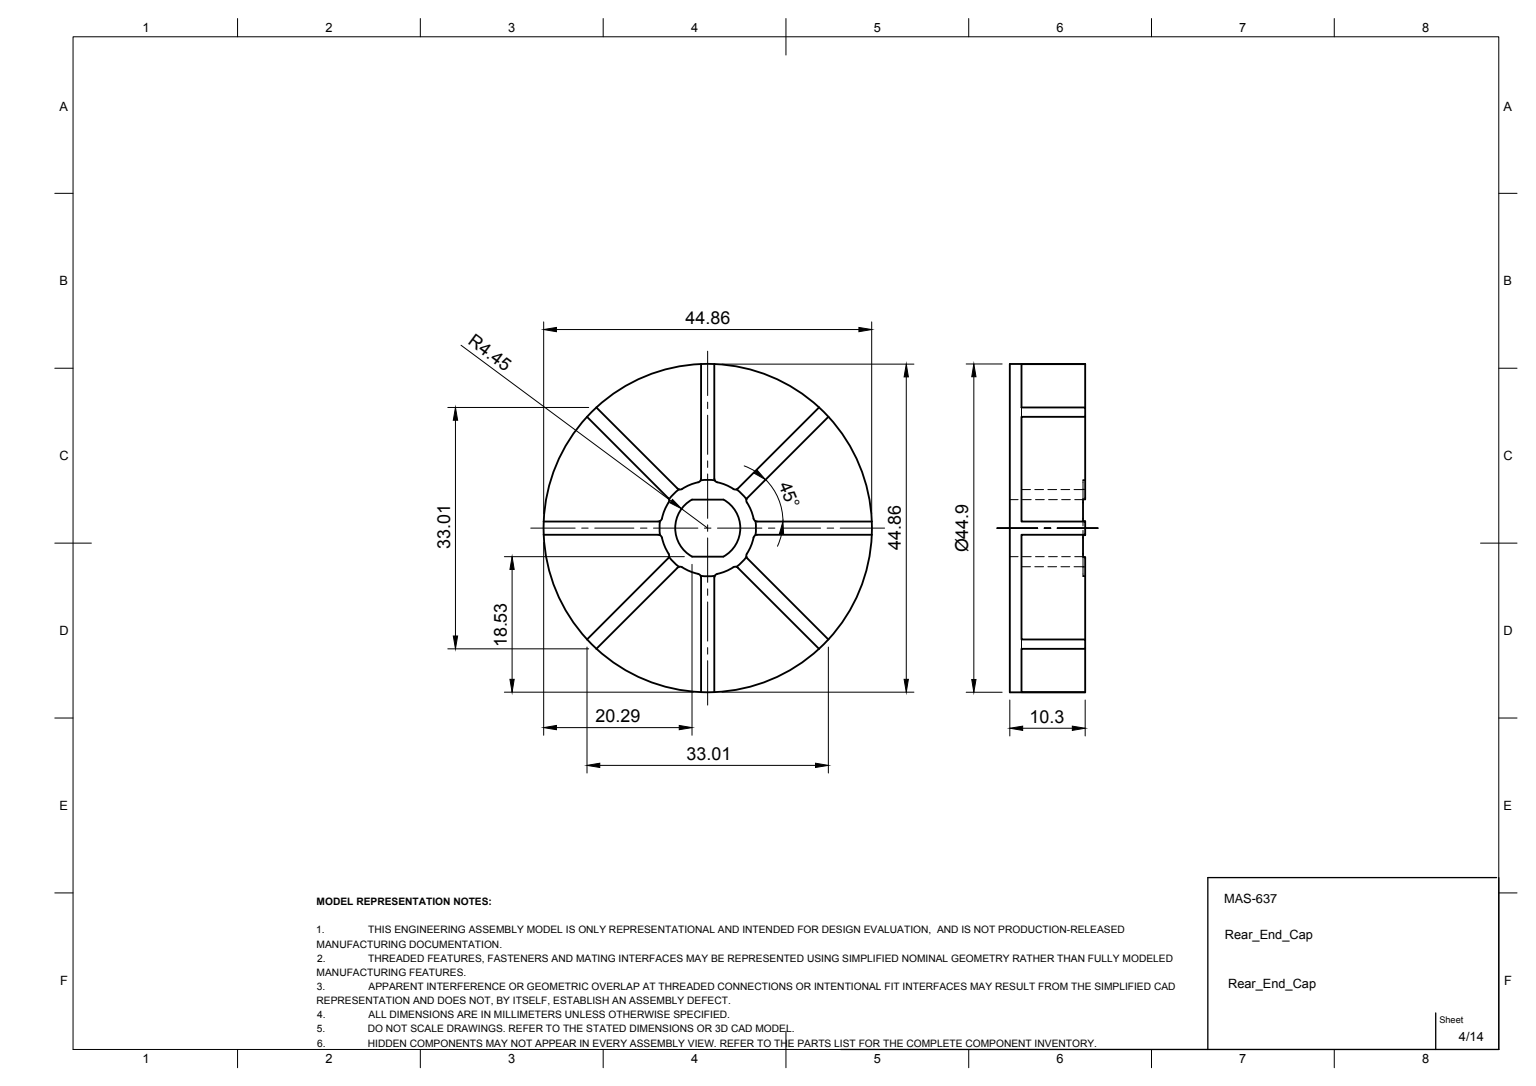
ISO-10303-21;
HEADER;
FILE_DESCRIPTION((''),'2;1');
FILE_NAME('Rear_End_Cap.step','2026-10-09T10:11:57-07:00',(''),(''),'','','');
FILE_SCHEMA (('AUTOMOTIVE_DESIGN { 1 0 10303 214 3 1 1 }'));
ENDSEC;
DATA;
#10=MECHANICAL_DESIGN_GEOMETRIC_PRESENTATION_REPRESENTATION('',(#124),#13510);
#94=SHAPE_REPRESENTATION_RELATIONSHIP('SRR','None',#13564,#109) ;
#109=ADVANCED_BREP_SHAPE_REPRESENTATION('',(#156),#13496) ;
#124=STYLED_ITEM('',(#13648),#156) ;
#156=MANIFOLD_SOLID_BREP('Body1',#7373) ;
#215=FACE_BOUND('',#1218,.T.) ;
#216=FACE_BOUND('',#1281,.T.) ;
#288=PLANE('',#7723) ;
#289=PLANE('',#7727) ;
#290=PLANE('',#7746) ;
#291=PLANE('',#7747) ;
#292=PLANE('',#7751) ;
#293=PLANE('',#7752) ;
#294=PLANE('',#7753) ;
#295=PLANE('',#7756) ;
#296=PLANE('',#7760) ;
#297=PLANE('',#7761) ;
#298=PLANE('',#7762) ;
#299=PLANE('',#7763) ;
#300=PLANE('',#7766) ;
#301=PLANE('',#7769) ;
#302=PLANE('',#7860) ;
#303=PLANE('',#7861) ;
#304=PLANE('',#7862) ;
#305=PLANE('',#7863) ;
#306=PLANE('',#7864) ;
#307=PLANE('',#7865) ;
#308=PLANE('',#7866) ;
#309=PLANE('',#7867) ;
#310=PLANE('',#7868) ;
#311=PLANE('',#7869) ;
#312=PLANE('',#7870) ;
#313=PLANE('',#7877) ;
#314=PLANE('',#7878) ;
#315=PLANE('',#7879) ;
#316=PLANE('',#7880) ;
#317=PLANE('',#7881) ;
#318=PLANE('',#7882) ;
#319=PLANE('',#7883) ;
#320=PLANE('',#7884) ;
#321=PLANE('',#7885) ;
#322=PLANE('',#7887) ;
#323=PLANE('',#7892) ;
#566=CYLINDRICAL_SURFACE('',#7720,6.6) ;
#567=CYLINDRICAL_SURFACE('',#7728,22.45) ;
#568=CYLINDRICAL_SURFACE('',#7757,0.5) ;
#569=CYLINDRICAL_SURFACE('',#7764,4.45) ;
#570=CYLINDRICAL_SURFACE('',#7767,4.45) ;
#571=CYLINDRICAL_SURFACE('',#7770,6.6) ;
#572=CYLINDRICAL_SURFACE('',#7773,0.5) ;
#573=CYLINDRICAL_SURFACE('',#7777,6.4) ;
#574=CYLINDRICAL_SURFACE('',#7780,0.5) ;
#575=CYLINDRICAL_SURFACE('',#7784,6.4) ;
#576=CYLINDRICAL_SURFACE('',#7787,0.5) ;
#577=CYLINDRICAL_SURFACE('',#7791,6.4) ;
#578=CYLINDRICAL_SURFACE('',#7794,0.5) ;
#579=CYLINDRICAL_SURFACE('',#7798,6.4) ;
#580=CYLINDRICAL_SURFACE('',#7801,0.5) ;
#581=CYLINDRICAL_SURFACE('',#7805,6.4) ;
#582=CYLINDRICAL_SURFACE('',#7808,0.5) ;
#583=CYLINDRICAL_SURFACE('',#7812,6.4) ;
#584=CYLINDRICAL_SURFACE('',#7815,6.6) ;
#585=CYLINDRICAL_SURFACE('',#7818,6.6) ;
#586=CYLINDRICAL_SURFACE('',#7821,6.6) ;
#587=CYLINDRICAL_SURFACE('',#7824,6.6) ;
#588=CYLINDRICAL_SURFACE('',#7827,6.6) ;
#589=CYLINDRICAL_SURFACE('',#7830,6.6) ;
#590=CYLINDRICAL_SURFACE('',#7833,6.4) ;
#591=CYLINDRICAL_SURFACE('',#7836,0.5) ;
#592=CYLINDRICAL_SURFACE('',#7840,0.5) ;
#593=CYLINDRICAL_SURFACE('',#7844,0.5) ;
#594=CYLINDRICAL_SURFACE('',#7848,0.5) ;
#595=CYLINDRICAL_SURFACE('',#7852,0.5) ;
#596=CYLINDRICAL_SURFACE('',#7856,0.5) ;
#597=CYLINDRICAL_SURFACE('',#7871,0.5) ;
#598=CYLINDRICAL_SURFACE('',#7875,6.4) ;
#599=CYLINDRICAL_SURFACE('',#7888,0.5) ;
#600=CYLINDRICAL_SURFACE('',#7890,0.5) ;
#733=FACE_OUTER_BOUND('',#1209,.T.) ;
#734=FACE_OUTER_BOUND('',#1210,.T.) ;
#735=FACE_OUTER_BOUND('',#1211,.T.) ;
#736=FACE_OUTER_BOUND('',#1212,.T.) ;
#737=FACE_OUTER_BOUND('',#1213,.T.) ;
#738=FACE_OUTER_BOUND('',#1214,.T.) ;
#739=FACE_OUTER_BOUND('',#1215,.T.) ;
#740=FACE_OUTER_BOUND('',#1216,.T.) ;
#741=FACE_OUTER_BOUND('',#1217,.T.) ;
#742=FACE_OUTER_BOUND('',#1219,.T.) ;
#743=FACE_OUTER_BOUND('',#1220,.T.) ;
#744=FACE_OUTER_BOUND('',#1221,.T.) ;
#745=FACE_OUTER_BOUND('',#1222,.T.) ;
#746=FACE_OUTER_BOUND('',#1223,.T.) ;
#747=FACE_OUTER_BOUND('',#1224,.T.) ;
#748=FACE_OUTER_BOUND('',#1225,.T.) ;
#749=FACE_OUTER_BOUND('',#1226,.T.) ;
#750=FACE_OUTER_BOUND('',#1227,.T.) ;
#751=FACE_OUTER_BOUND('',#1228,.T.) ;
#752=FACE_OUTER_BOUND('',#1229,.T.) ;
#753=FACE_OUTER_BOUND('',#1230,.T.) ;
#754=FACE_OUTER_BOUND('',#1231,.T.) ;
#755=FACE_OUTER_BOUND('',#1232,.T.) ;
#756=FACE_OUTER_BOUND('',#1233,.T.) ;
#757=FACE_OUTER_BOUND('',#1234,.T.) ;
#758=FACE_OUTER_BOUND('',#1235,.T.) ;
#759=FACE_OUTER_BOUND('',#1236,.T.) ;
#760=FACE_OUTER_BOUND('',#1237,.T.) ;
#761=FACE_OUTER_BOUND('',#1238,.T.) ;
#762=FACE_OUTER_BOUND('',#1239,.T.) ;
#763=FACE_OUTER_BOUND('',#1240,.T.) ;
#764=FACE_OUTER_BOUND('',#1241,.T.) ;
#765=FACE_OUTER_BOUND('',#1242,.T.) ;
#766=FACE_OUTER_BOUND('',#1243,.T.) ;
#767=FACE_OUTER_BOUND('',#1244,.T.) ;
#768=FACE_OUTER_BOUND('',#1245,.T.) ;
#769=FACE_OUTER_BOUND('',#1246,.T.) ;
#770=FACE_OUTER_BOUND('',#1247,.T.) ;
#771=FACE_OUTER_BOUND('',#1248,.T.) ;
#772=FACE_OUTER_BOUND('',#1249,.T.) ;
#773=FACE_OUTER_BOUND('',#1250,.T.) ;
#774=FACE_OUTER_BOUND('',#1251,.T.) ;
#775=FACE_OUTER_BOUND('',#1252,.T.) ;
#776=FACE_OUTER_BOUND('',#1253,.T.) ;
#777=FACE_OUTER_BOUND('',#1254,.T.) ;
#778=FACE_OUTER_BOUND('',#1255,.T.) ;
#779=FACE_OUTER_BOUND('',#1256,.T.) ;
#780=FACE_OUTER_BOUND('',#1257,.T.) ;
#781=FACE_OUTER_BOUND('',#1258,.T.) ;
#782=FACE_OUTER_BOUND('',#1259,.T.) ;
#783=FACE_OUTER_BOUND('',#1260,.T.) ;
#784=FACE_OUTER_BOUND('',#1261,.T.) ;
#785=FACE_OUTER_BOUND('',#1262,.T.) ;
#786=FACE_OUTER_BOUND('',#1263,.T.) ;
#787=FACE_OUTER_BOUND('',#1264,.T.) ;
#788=FACE_OUTER_BOUND('',#1265,.T.) ;
#789=FACE_OUTER_BOUND('',#1266,.T.) ;
#790=FACE_OUTER_BOUND('',#1267,.T.) ;
#791=FACE_OUTER_BOUND('',#1268,.T.) ;
#792=FACE_OUTER_BOUND('',#1269,.T.) ;
#793=FACE_OUTER_BOUND('',#1270,.T.) ;
#794=FACE_OUTER_BOUND('',#1271,.T.) ;
#795=FACE_OUTER_BOUND('',#1272,.T.) ;
#796=FACE_OUTER_BOUND('',#1273,.T.) ;
#797=FACE_OUTER_BOUND('',#1274,.T.) ;
#798=FACE_OUTER_BOUND('',#1275,.T.) ;
#799=FACE_OUTER_BOUND('',#1276,.T.) ;
#800=FACE_OUTER_BOUND('',#1277,.T.) ;
#801=FACE_OUTER_BOUND('',#1278,.T.) ;
#802=FACE_OUTER_BOUND('',#1279,.T.) ;
#803=FACE_OUTER_BOUND('',#1280,.T.) ;
#1209=EDGE_LOOP('',(#5152,#5153,#5154,#5155)) ;
#1210=EDGE_LOOP('',(#5156,#5157,#5158,#5159,#5160,#5161)) ;
#1211=EDGE_LOOP('',(#5162,#5163,#5164,#5165)) ;
#1212=EDGE_LOOP('',(#5166,#5167,#5168,#5169,#5170,#5171,#5172,#5173,#5174,
#5175,#5176,#5177,#5178,#5179,#5180,#5181,#5182,#5183,#5184,#5185,#5186,
#5187,#5188,#5189,#5190,#5191,#5192,#5193,#5194,#5195,#5196,#5197,#5198,
#5199,#5200,#5201)) ;
#1213=EDGE_LOOP('',(#5202,#5203,#5204,#5205)) ;
#1214=EDGE_LOOP('',(#5206,#5207,#5208,#5209,#5210,#5211)) ;
#1215=EDGE_LOOP('',(#5212,#5213,#5214,#5215)) ;
#1216=EDGE_LOOP('',(#5216,#5217,#5218,#5219)) ;
#1217=EDGE_LOOP('',(#5220)) ;
#1218=EDGE_LOOP('',(#5221,#5222,#5223,#5224)) ;
#1219=EDGE_LOOP('',(#5225,#5226,#5227,#5228)) ;
#1220=EDGE_LOOP('',(#5229,#5230,#5231,#5232,#5233,#5234)) ;
#1221=EDGE_LOOP('',(#5235,#5236,#5237,#5238)) ;
#1222=EDGE_LOOP('',(#5239,#5240,#5241,#5242)) ;
#1223=EDGE_LOOP('',(#5243,#5244,#5245,#5246)) ;
#1224=EDGE_LOOP('',(#5247,#5248,#5249,#5250)) ;
#1225=EDGE_LOOP('',(#5251,#5252,#5253,#5254)) ;
#1226=EDGE_LOOP('',(#5255,#5256,#5257,#5258)) ;
#1227=EDGE_LOOP('',(#5259,#5260,#5261,#5262)) ;
#1228=EDGE_LOOP('',(#5263,#5264,#5265,#5266)) ;
#1229=EDGE_LOOP('',(#5267,#5268,#5269,#5270)) ;
#1230=EDGE_LOOP('',(#5271,#5272,#5273,#5274,#5275,#5276)) ;
#1231=EDGE_LOOP('',(#5277,#5278,#5279,#5280)) ;
#1232=EDGE_LOOP('',(#5281,#5282,#5283,#5284,#5285,#5286)) ;
#1233=EDGE_LOOP('',(#5287,#5288,#5289,#5290)) ;
#1234=EDGE_LOOP('',(#5291,#5292,#5293,#5294,#5295,#5296)) ;
#1235=EDGE_LOOP('',(#5297,#5298,#5299,#5300)) ;
#1236=EDGE_LOOP('',(#5301,#5302,#5303,#5304,#5305,#5306)) ;
#1237=EDGE_LOOP('',(#5307,#5308,#5309,#5310)) ;
#1238=EDGE_LOOP('',(#5311,#5312,#5313,#5314,#5315,#5316)) ;
#1239=EDGE_LOOP('',(#5317,#5318,#5319,#5320)) ;
#1240=EDGE_LOOP('',(#5321,#5322,#5323,#5324,#5325,#5326)) ;
#1241=EDGE_LOOP('',(#5327,#5328,#5329,#5330)) ;
#1242=EDGE_LOOP('',(#5331,#5332,#5333,#5334)) ;
#1243=EDGE_LOOP('',(#5335,#5336,#5337,#5338)) ;
#1244=EDGE_LOOP('',(#5339,#5340,#5341,#5342)) ;
#1245=EDGE_LOOP('',(#5343,#5344,#5345,#5346)) ;
#1246=EDGE_LOOP('',(#5347,#5348,#5349,#5350)) ;
#1247=EDGE_LOOP('',(#5351,#5352,#5353,#5354)) ;
#1248=EDGE_LOOP('',(#5355,#5356,#5357,#5358)) ;
#1249=EDGE_LOOP('',(#5359,#5360,#5361,#5362,#5363,#5364)) ;
#1250=EDGE_LOOP('',(#5365,#5366,#5367,#5368,#5369,#5370)) ;
#1251=EDGE_LOOP('',(#5371,#5372,#5373,#5374,#5375,#5376)) ;
#1252=EDGE_LOOP('',(#5377,#5378,#5379,#5380,#5381,#5382)) ;
#1253=EDGE_LOOP('',(#5383,#5384,#5385,#5386,#5387,#5388)) ;
#1254=EDGE_LOOP('',(#5389,#5390,#5391,#5392,#5393,#5394)) ;
#1255=EDGE_LOOP('',(#5395,#5396,#5397,#5398)) ;
#1256=EDGE_LOOP('',(#5399,#5400,#5401,#5402,#5403,#5404)) ;
#1257=EDGE_LOOP('',(#5405,#5406,#5407,#5408,#5409,#5410)) ;
#1258=EDGE_LOOP('',(#5411,#5412,#5413,#5414)) ;
#1259=EDGE_LOOP('',(#5415,#5416,#5417,#5418,#5419,#5420)) ;
#1260=EDGE_LOOP('',(#5421,#5422,#5423,#5424,#5425,#5426)) ;
#1261=EDGE_LOOP('',(#5427,#5428,#5429,#5430)) ;
#1262=EDGE_LOOP('',(#5431,#5432,#5433,#5434,#5435,#5436)) ;
#1263=EDGE_LOOP('',(#5437,#5438,#5439,#5440,#5441,#5442)) ;
#1264=EDGE_LOOP('',(#5443,#5444,#5445,#5446)) ;
#1265=EDGE_LOOP('',(#5447,#5448,#5449,#5450,#5451,#5452)) ;
#1266=EDGE_LOOP('',(#5453,#5454,#5455,#5456,#5457,#5458)) ;
#1267=EDGE_LOOP('',(#5459,#5460,#5461,#5462)) ;
#1268=EDGE_LOOP('',(#5463,#5464,#5465,#5466,#5467,#5468)) ;
#1269=EDGE_LOOP('',(#5469,#5470,#5471,#5472,#5473,#5474,#5475)) ;
#1270=EDGE_LOOP('',(#5476,#5477,#5478,#5479,#5480,#5481)) ;
#1271=EDGE_LOOP('',(#5482,#5483,#5484,#5485)) ;
#1272=EDGE_LOOP('',(#5486,#5487,#5488,#5489,#5490,#5491)) ;
#1273=EDGE_LOOP('',(#5492,#5493,#5494,#5495,#5496,#5497)) ;
#1274=EDGE_LOOP('',(#5498,#5499,#5500,#5501)) ;
#1275=EDGE_LOOP('',(#5502,#5503,#5504,#5505,#5506,#5507)) ;
#1276=EDGE_LOOP('',(#5508,#5509,#5510,#5511,#5512,#5513)) ;
#1277=EDGE_LOOP('',(#5514,#5515,#5516,#5517)) ;
#1278=EDGE_LOOP('',(#5518,#5519,#5520,#5521,#5522,#5523)) ;
#1279=EDGE_LOOP('',(#5524,#5525,#5526,#5527,#5528,#5529)) ;
#1280=EDGE_LOOP('',(#5530,#5531,#5532,#5533,#5534,#5535,#5536,#5537,#5538,
#5539,#5540,#5541,#5542,#5543,#5544,#5545,#5546,#5547,#5548,#5549,#5550,
#5551,#5552,#5553,#5554,#5555,#5556,#5557,#5558,#5559,#5560,#5561)) ;
#1281=EDGE_LOOP('',(#5562,#5563,#5564,#5565)) ;
#1717=LINE('',#11554,#2211) ;
#1718=LINE('',#11558,#2212) ;
#1719=LINE('',#11564,#2213) ;
#1720=LINE('',#11568,#2214) ;
#1721=LINE('',#11572,#2215) ;
#1722=LINE('',#11574,#2216) ;
#1723=LINE('',#11575,#2217) ;
#1724=LINE('',#11581,#2218) ;
#1725=LINE('',#11585,#2219) ;
#1726=LINE('',#11588,#2220) ;
#1727=LINE('',#11592,#2221) ;
#1728=LINE('',#11596,#2222) ;
#1729=LINE('',#11600,#2223) ;
#1730=LINE('',#11604,#2224) ;
#1731=LINE('',#11608,#2225) ;
#1732=LINE('',#11612,#2226) ;
#1733=LINE('',#11616,#2227) ;
#1734=LINE('',#11620,#2228) ;
#1735=LINE('',#11624,#2229) ;
#1736=LINE('',#11628,#2230) ;
#1737=LINE('',#11632,#2231) ;
#1738=LINE('',#11636,#2232) ;
#1739=LINE('',#11639,#2233) ;
#1740=LINE('',#11643,#2234) ;
#1741=LINE('',#11644,#2235) ;
#1742=LINE('',#11651,#2236) ;
#1743=LINE('',#11655,#2237) ;
#1744=LINE('',#11656,#2238) ;
#1745=LINE('',#11660,#2239) ;
#1746=LINE('',#11661,#2240) ;
#1747=LINE('',#11662,#2241) ;
#1748=LINE('',#11666,#2242) ;
#1749=LINE('',#11670,#2243) ;
#1750=LINE('',#11675,#2244) ;
#1751=LINE('',#11676,#2245) ;
#1752=LINE('',#11677,#2246) ;
#1753=LINE('',#11683,#2247) ;
#1754=LINE('',#11685,#2248) ;
#1755=LINE('',#11689,#2249) ;
#1756=LINE('',#11690,#2250) ;
#1757=LINE('',#11691,#2251) ;
#1758=LINE('',#11695,#2252) ;
#1759=LINE('',#11696,#2253) ;
#1760=LINE('',#11697,#2254) ;
#1761=LINE('',#11701,#2255) ;
#1762=LINE('',#11702,#2256) ;
#1763=LINE('',#11703,#2257) ;
#1764=LINE('',#11707,#2258) ;
#1765=LINE('',#11708,#2259) ;
#1766=LINE('',#11709,#2260) ;
#1767=LINE('',#11714,#2261) ;
#1768=LINE('',#11715,#2262) ;
#1769=LINE('',#11718,#2263) ;
#1770=LINE('',#11719,#2264) ;
#1771=LINE('',#11723,#2265) ;
#1772=LINE('',#11725,#2266) ;
#1773=LINE('',#11731,#2267) ;
#1774=LINE('',#11735,#2268) ;
#1775=LINE('',#11739,#2269) ;
#1776=LINE('',#11743,#2270) ;
#1777=LINE('',#11750,#2271) ;
#1778=LINE('',#11753,#2272) ;
#1779=LINE('',#11757,#2273) ;
#1780=LINE('',#11762,#2274) ;
#1781=LINE('',#11769,#2275) ;
#1782=LINE('',#11772,#2276) ;
#1783=LINE('',#11776,#2277) ;
#1784=LINE('',#11781,#2278) ;
#1785=LINE('',#11788,#2279) ;
#1786=LINE('',#11791,#2280) ;
#1787=LINE('',#11795,#2281) ;
#1788=LINE('',#11800,#2282) ;
#1789=LINE('',#11807,#2283) ;
#1790=LINE('',#11810,#2284) ;
#1791=LINE('',#11814,#2285) ;
#1792=LINE('',#11819,#2286) ;
#1793=LINE('',#11826,#2287) ;
#1794=LINE('',#11829,#2288) ;
#1795=LINE('',#11833,#2289) ;
#1796=LINE('',#11838,#2290) ;
#1797=LINE('',#11845,#2291) ;
#1798=LINE('',#11848,#2292) ;
#1799=LINE('',#11853,#2293) ;
#1800=LINE('',#11859,#2294) ;
#1801=LINE('',#11865,#2295) ;
#1802=LINE('',#11871,#2296) ;
#1803=LINE('',#11877,#2297) ;
#1804=LINE('',#11883,#2298) ;
#1805=LINE('',#11889,#2299) ;
#1806=LINE('',#11896,#2300) ;
#1807=LINE('',#11919,#2301) ;
#1808=LINE('',#11920,#2302) ;
#1809=LINE('',#11923,#2303) ;
#1810=LINE('',#11925,#2304) ;
#1811=LINE('',#11928,#2305) ;
#1812=LINE('',#11930,#2306) ;
#1813=LINE('',#11933,#2307) ;
#1814=LINE('',#11935,#2308) ;
#1815=LINE('',#11944,#2309) ;
#1816=LINE('',#11946,#2310) ;
#1817=LINE('',#11949,#2311) ;
#1818=LINE('',#11951,#2312) ;
#1819=LINE('',#11954,#2313) ;
#1820=LINE('',#11956,#2314) ;
#1821=LINE('',#11960,#2315) ;
#2211=VECTOR('',#8937,1.) ;
#2212=VECTOR('',#8940,1.) ;
#2213=VECTOR('',#8947,1.00000000000064) ;
#2214=VECTOR('',#8950,1.00000000000064) ;
#2215=VECTOR('',#8955,1.) ;
#2216=VECTOR('',#8956,1.00000000000064) ;
#2217=VECTOR('',#8957,1.) ;
#2218=VECTOR('',#8962,1.) ;
#2219=VECTOR('',#8965,1.) ;
#2220=VECTOR('',#8968,1.) ;
#2221=VECTOR('',#8971,1.) ;
#2222=VECTOR('',#8974,1.) ;
#2223=VECTOR('',#8977,1.) ;
#2224=VECTOR('',#8980,1.) ;
#2225=VECTOR('',#8983,1.) ;
#2226=VECTOR('',#8986,1.) ;
#2227=VECTOR('',#8989,1.) ;
#2228=VECTOR('',#8992,1.) ;
#2229=VECTOR('',#8995,1.) ;
#2230=VECTOR('',#8998,1.) ;
#2231=VECTOR('',#9001,1.) ;
#2232=VECTOR('',#9004,1.) ;
#2233=VECTOR('',#9007,22.45) ;
#2234=VECTOR('',#9012,1.) ;
#2235=VECTOR('',#9013,1.00000000000064) ;
#2236=VECTOR('',#9020,1.) ;
#2237=VECTOR('',#9025,1.) ;
#2238=VECTOR('',#9026,1.) ;
#2239=VECTOR('',#9029,1.) ;
#2240=VECTOR('',#9030,1.00000000000064) ;
#2241=VECTOR('',#9031,1.00000000000064) ;
#2242=VECTOR('',#9034,1.) ;
#2243=VECTOR('',#9037,1.) ;
#2244=VECTOR('',#9042,1.) ;
#2245=VECTOR('',#9043,1.) ;
#2246=VECTOR('',#9044,1.) ;
#2247=VECTOR('',#9049,1.) ;
#2248=VECTOR('',#9052,1.) ;
#2249=VECTOR('',#9055,1.) ;
#2250=VECTOR('',#9056,1.) ;
#2251=VECTOR('',#9057,1.) ;
#2252=VECTOR('',#9060,1.) ;
#2253=VECTOR('',#9061,1.00000000000064) ;
#2254=VECTOR('',#9062,1.00000000000064) ;
#2255=VECTOR('',#9065,1.) ;
#2256=VECTOR('',#9066,1.) ;
#2257=VECTOR('',#9067,1.) ;
#2258=VECTOR('',#9070,1.) ;
#2259=VECTOR('',#9071,1.00000000000064) ;
#2260=VECTOR('',#9072,1.00000000000064) ;
#2261=VECTOR('',#9077,1.) ;
#2262=VECTOR('',#9078,1.) ;
#2263=VECTOR('',#9081,1.) ;
#2264=VECTOR('',#9082,1.) ;
#2265=VECTOR('',#9087,1.) ;
#2266=VECTOR('',#9090,1.) ;
#2267=VECTOR('',#9097,1.) ;
#2268=VECTOR('',#9100,1.) ;
#2269=VECTOR('',#9103,1.) ;
#2270=VECTOR('',#9106,1.) ;
#2271=VECTOR('',#9113,1.) ;
#2272=VECTOR('',#9116,1.) ;
#2273=VECTOR('',#9119,1.) ;
#2274=VECTOR('',#9124,1.) ;
#2275=VECTOR('',#9131,1.) ;
#2276=VECTOR('',#9134,1.) ;
#2277=VECTOR('',#9137,1.) ;
#2278=VECTOR('',#9142,1.) ;
#2279=VECTOR('',#9149,1.) ;
#2280=VECTOR('',#9152,1.) ;
#2281=VECTOR('',#9155,1.) ;
#2282=VECTOR('',#9160,1.) ;
#2283=VECTOR('',#9167,1.) ;
#2284=VECTOR('',#9170,1.) ;
#2285=VECTOR('',#9173,1.) ;
#2286=VECTOR('',#9178,1.) ;
#2287=VECTOR('',#9185,1.) ;
#2288=VECTOR('',#9188,1.) ;
#2289=VECTOR('',#9191,1.) ;
#2290=VECTOR('',#9196,1.) ;
#2291=VECTOR('',#9203,1.) ;
#2292=VECTOR('',#9206,1.) ;
#2293=VECTOR('',#9211,1.) ;
#2294=VECTOR('',#9218,1.) ;
#2295=VECTOR('',#9225,1.) ;
#2296=VECTOR('',#9232,1.) ;
#2297=VECTOR('',#9239,1.) ;
#2298=VECTOR('',#9246,1.) ;
#2299=VECTOR('',#9253,1.) ;
#2300=VECTOR('',#9262,1.) ;
#2301=VECTOR('',#9307,1.00000000000064) ;
#2302=VECTOR('',#9308,1.00000000000064) ;
#2303=VECTOR('',#9313,1.) ;
#2304=VECTOR('',#9316,1.) ;
#2305=VECTOR('',#9321,1.00000000000064) ;
#2306=VECTOR('',#9324,1.00000000000064) ;
#2307=VECTOR('',#9329,1.) ;
#2308=VECTOR('',#9332,1.) ;
#2309=VECTOR('',#9347,1.) ;
#2310=VECTOR('',#9350,1.) ;
#2311=VECTOR('',#9355,1.00000000000064) ;
#2312=VECTOR('',#9358,1.00000000000064) ;
#2313=VECTOR('',#9363,1.) ;
#2314=VECTOR('',#9366,1.) ;
#2315=VECTOR('',#9373,1.) ;
#2713=CIRCLE('',#7721,6.6) ;
#2714=CIRCLE('',#7722,6.6) ;
#2715=CIRCLE('',#7724,0.5) ;
#2716=CIRCLE('',#7725,22.45) ;
#2717=CIRCLE('',#7726,0.5) ;
#2718=CIRCLE('',#7729,22.45) ;
#2719=CIRCLE('',#7730,22.45) ;
#2720=CIRCLE('',#7731,22.45) ;
#2721=CIRCLE('',#7732,22.45) ;
#2722=CIRCLE('',#7733,22.45) ;
#2723=CIRCLE('',#7734,22.45) ;
#2724=CIRCLE('',#7735,22.45) ;
#2725=CIRCLE('',#7736,22.45) ;
#2726=CIRCLE('',#7737,22.45) ;
#2727=CIRCLE('',#7738,22.45) ;
#2728=CIRCLE('',#7739,22.45) ;
#2729=CIRCLE('',#7740,22.45) ;
#2730=CIRCLE('',#7741,22.45) ;
#2731=CIRCLE('',#7742,22.45) ;
#2732=CIRCLE('',#7743,22.45) ;
#2733=CIRCLE('',#7744,22.45) ;
#2734=CIRCLE('',#7745,22.45) ;
#2735=CIRCLE('',#7748,6.4) ;
#2736=CIRCLE('',#7749,0.5) ;
#2737=CIRCLE('',#7750,0.5) ;
#2738=CIRCLE('',#7754,4.45) ;
#2739=CIRCLE('',#7755,4.45) ;
#2740=CIRCLE('',#7758,0.5) ;
#2741=CIRCLE('',#7759,0.5) ;
#2742=CIRCLE('',#7765,4.45) ;
#2743=CIRCLE('',#7768,4.45) ;
#2744=CIRCLE('',#7771,6.6) ;
#2745=CIRCLE('',#7772,6.6) ;
#2746=CIRCLE('',#7774,0.5) ;
#2747=CIRCLE('',#7775,0.5) ;
#2748=CIRCLE('',#7776,0.5) ;
#2749=CIRCLE('',#7778,6.4) ;
#2750=CIRCLE('',#7779,6.4) ;
#2751=CIRCLE('',#7781,0.5) ;
#2752=CIRCLE('',#7782,0.5) ;
#2753=CIRCLE('',#7783,0.5) ;
#2754=CIRCLE('',#7785,6.4) ;
#2755=CIRCLE('',#7786,6.4) ;
#2756=CIRCLE('',#7788,0.5) ;
#2757=CIRCLE('',#7789,0.5) ;
#2758=CIRCLE('',#7790,0.5) ;
#2759=CIRCLE('',#7792,6.4) ;
#2760=CIRCLE('',#7793,6.4) ;
#2761=CIRCLE('',#7795,0.5) ;
#2762=CIRCLE('',#7796,0.5) ;
#2763=CIRCLE('',#7797,0.5) ;
#2764=CIRCLE('',#7799,6.4) ;
#2765=CIRCLE('',#7800,6.4) ;
#2766=CIRCLE('',#7802,0.5) ;
#2767=CIRCLE('',#7803,0.5) ;
#2768=CIRCLE('',#7804,0.5) ;
#2769=CIRCLE('',#7806,6.4) ;
#2770=CIRCLE('',#7807,6.4) ;
#2771=CIRCLE('',#7809,0.5) ;
#2772=CIRCLE('',#7810,0.5) ;
#2773=CIRCLE('',#7811,0.5) ;
#2774=CIRCLE('',#7813,6.4) ;
#2775=CIRCLE('',#7814,6.4) ;
#2776=CIRCLE('',#7816,6.6) ;
#2777=CIRCLE('',#7817,6.6) ;
#2778=CIRCLE('',#7819,6.6) ;
#2779=CIRCLE('',#7820,6.6) ;
#2780=CIRCLE('',#7822,6.6) ;
#2781=CIRCLE('',#7823,6.6) ;
#2782=CIRCLE('',#7825,6.6) ;
#2783=CIRCLE('',#7826,6.6) ;
#2784=CIRCLE('',#7828,6.6) ;
#2785=CIRCLE('',#7829,6.6) ;
#2786=CIRCLE('',#7831,6.6) ;
#2787=CIRCLE('',#7832,6.6) ;
#2788=CIRCLE('',#7834,6.4) ;
#2789=CIRCLE('',#7835,6.4) ;
#2790=CIRCLE('',#7837,0.5) ;
#2791=CIRCLE('',#7838,0.5) ;
#2792=CIRCLE('',#7839,0.5) ;
#2793=CIRCLE('',#7841,0.5) ;
#2794=CIRCLE('',#7842,0.5) ;
#2795=CIRCLE('',#7843,0.5) ;
#2796=CIRCLE('',#7845,0.5) ;
#2797=CIRCLE('',#7846,0.5) ;
#2798=CIRCLE('',#7847,0.5) ;
#2799=CIRCLE('',#7849,0.5) ;
#2800=CIRCLE('',#7850,0.5) ;
#2801=CIRCLE('',#7851,0.5) ;
#2802=CIRCLE('',#7853,0.5) ;
#2803=CIRCLE('',#7854,0.5) ;
#2804=CIRCLE('',#7855,0.5) ;
#2805=CIRCLE('',#7857,0.5) ;
#2806=CIRCLE('',#7858,0.5) ;
#2807=CIRCLE('',#7859,0.5) ;
#2808=CIRCLE('',#7872,0.5) ;
#2809=CIRCLE('',#7873,0.5) ;
#2810=CIRCLE('',#7874,0.5) ;
#2811=CIRCLE('',#7876,6.4) ;
#2812=CIRCLE('',#7886,0.5) ;
#2813=CIRCLE('',#7889,0.5) ;
#2814=CIRCLE('',#7891,0.5) ;
#3247=VERTEX_POINT('',#11552) ;
#3248=VERTEX_POINT('',#11553) ;
#3249=VERTEX_POINT('',#11555) ;
#3250=VERTEX_POINT('',#11557) ;
#3251=VERTEX_POINT('',#11561) ;
#3252=VERTEX_POINT('',#11563) ;
#3253=VERTEX_POINT('',#11565) ;
#3254=VERTEX_POINT('',#11567) ;
#3255=VERTEX_POINT('',#11571) ;
#3256=VERTEX_POINT('',#11573) ;
#3257=VERTEX_POINT('',#11577) ;
#3258=VERTEX_POINT('',#11578) ;
#3259=VERTEX_POINT('',#11580) ;
#3260=VERTEX_POINT('',#11582) ;
#3261=VERTEX_POINT('',#11584) ;
#3262=VERTEX_POINT('',#11586) ;
#3263=VERTEX_POINT('',#11589) ;
#3264=VERTEX_POINT('',#11591) ;
#3265=VERTEX_POINT('',#11593) ;
#3266=VERTEX_POINT('',#11595) ;
#3267=VERTEX_POINT('',#11597) ;
#3268=VERTEX_POINT('',#11599) ;
#3269=VERTEX_POINT('',#11601) ;
#3270=VERTEX_POINT('',#11603) ;
#3271=VERTEX_POINT('',#11605) ;
#3272=VERTEX_POINT('',#11607) ;
#3273=VERTEX_POINT('',#11609) ;
#3274=VERTEX_POINT('',#11611) ;
#3275=VERTEX_POINT('',#11613) ;
#3276=VERTEX_POINT('',#11615) ;
#3277=VERTEX_POINT('',#11617) ;
#3278=VERTEX_POINT('',#11619) ;
#3279=VERTEX_POINT('',#11621) ;
#3280=VERTEX_POINT('',#11623) ;
#3281=VERTEX_POINT('',#11625) ;
#3282=VERTEX_POINT('',#11627) ;
#3283=VERTEX_POINT('',#11629) ;
#3284=VERTEX_POINT('',#11631) ;
#3285=VERTEX_POINT('',#11633) ;
#3286=VERTEX_POINT('',#11635) ;
#3287=VERTEX_POINT('',#11638) ;
#3288=VERTEX_POINT('',#11642) ;
#3289=VERTEX_POINT('',#11646) ;
#3290=VERTEX_POINT('',#11647) ;
#3291=VERTEX_POINT('',#11649) ;
#3292=VERTEX_POINT('',#11654) ;
#3293=VERTEX_POINT('',#11658) ;
#3294=VERTEX_POINT('',#11659) ;
#3295=VERTEX_POINT('',#11664) ;
#3296=VERTEX_POINT('',#11665) ;
#3297=VERTEX_POINT('',#11667) ;
#3298=VERTEX_POINT('',#11669) ;
#3299=VERTEX_POINT('',#11673) ;
#3300=VERTEX_POINT('',#11674) ;
#3301=VERTEX_POINT('',#11679) ;
#3302=VERTEX_POINT('',#11680) ;
#3303=VERTEX_POINT('',#11682) ;
#3304=VERTEX_POINT('',#11687) ;
#3305=VERTEX_POINT('',#11688) ;
#3306=VERTEX_POINT('',#11693) ;
#3307=VERTEX_POINT('',#11694) ;
#3308=VERTEX_POINT('',#11699) ;
#3309=VERTEX_POINT('',#11700) ;
#3310=VERTEX_POINT('',#11705) ;
#3311=VERTEX_POINT('',#11706) ;
#3312=VERTEX_POINT('',#11711) ;
#3313=VERTEX_POINT('',#11712) ;
#3314=VERTEX_POINT('',#11717) ;
#3315=VERTEX_POINT('',#11721) ;
#3316=VERTEX_POINT('',#11727) ;
#3317=VERTEX_POINT('',#11729) ;
#3318=VERTEX_POINT('',#11733) ;
#3319=VERTEX_POINT('',#11734) ;
#3320=VERTEX_POINT('',#11736) ;
#3321=VERTEX_POINT('',#11738) ;
#3322=VERTEX_POINT('',#11740) ;
#3323=VERTEX_POINT('',#11742) ;
#3324=VERTEX_POINT('',#11746) ;
#3325=VERTEX_POINT('',#11747) ;
#3326=VERTEX_POINT('',#11749) ;
#3327=VERTEX_POINT('',#11751) ;
#3328=VERTEX_POINT('',#11755) ;
#3329=VERTEX_POINT('',#11756) ;
#3330=VERTEX_POINT('',#11759) ;
#3331=VERTEX_POINT('',#11761) ;
#3332=VERTEX_POINT('',#11765) ;
#3333=VERTEX_POINT('',#11766) ;
#3334=VERTEX_POINT('',#11768) ;
#3335=VERTEX_POINT('',#11770) ;
#3336=VERTEX_POINT('',#11774) ;
#3337=VERTEX_POINT('',#11775) ;
#3338=VERTEX_POINT('',#11778) ;
#3339=VERTEX_POINT('',#11780) ;
#3340=VERTEX_POINT('',#11784) ;
#3341=VERTEX_POINT('',#11785) ;
#3342=VERTEX_POINT('',#11787) ;
#3343=VERTEX_POINT('',#11789) ;
#3344=VERTEX_POINT('',#11793) ;
#3345=VERTEX_POINT('',#11794) ;
#3346=VERTEX_POINT('',#11797) ;
#3347=VERTEX_POINT('',#11799) ;
#3348=VERTEX_POINT('',#11803) ;
#3349=VERTEX_POINT('',#11804) ;
#3350=VERTEX_POINT('',#11806) ;
#3351=VERTEX_POINT('',#11808) ;
#3352=VERTEX_POINT('',#11812) ;
#3353=VERTEX_POINT('',#11813) ;
#3354=VERTEX_POINT('',#11816) ;
#3355=VERTEX_POINT('',#11818) ;
#3356=VERTEX_POINT('',#11822) ;
#3357=VERTEX_POINT('',#11823) ;
#3358=VERTEX_POINT('',#11825) ;
#3359=VERTEX_POINT('',#11827) ;
#3360=VERTEX_POINT('',#11831) ;
#3361=VERTEX_POINT('',#11832) ;
#3362=VERTEX_POINT('',#11835) ;
#3363=VERTEX_POINT('',#11837) ;
#3364=VERTEX_POINT('',#11841) ;
#3365=VERTEX_POINT('',#11842) ;
#3366=VERTEX_POINT('',#11844) ;
#3367=VERTEX_POINT('',#11846) ;
#3368=VERTEX_POINT('',#11850) ;
#3369=VERTEX_POINT('',#11852) ;
#3370=VERTEX_POINT('',#11856) ;
#3371=VERTEX_POINT('',#11858) ;
#3372=VERTEX_POINT('',#11862) ;
#3373=VERTEX_POINT('',#11864) ;
#3374=VERTEX_POINT('',#11868) ;
#3375=VERTEX_POINT('',#11870) ;
#3376=VERTEX_POINT('',#11874) ;
#3377=VERTEX_POINT('',#11876) ;
#3378=VERTEX_POINT('',#11880) ;
#3379=VERTEX_POINT('',#11882) ;
#3380=VERTEX_POINT('',#11886) ;
#3381=VERTEX_POINT('',#11888) ;
#3382=VERTEX_POINT('',#11893) ;
#3383=VERTEX_POINT('',#11895) ;
#3384=VERTEX_POINT('',#11942) ;
#3963=EDGE_CURVE('',#3247,#3248,#1717,.T.) ;
#3964=EDGE_CURVE('',#3248,#3249,#2713,.T.) ;
#3965=EDGE_CURVE('',#3249,#3250,#1718,.F.) ;
#3966=EDGE_CURVE('',#3247,#3250,#2714,.T.) ;
#3967=EDGE_CURVE('',#3248,#3251,#2715,.F.) ;
#3968=EDGE_CURVE('',#3251,#3252,#1719,.F.) ;
#3969=EDGE_CURVE('',#3252,#3253,#2716,.T.) ;
#3970=EDGE_CURVE('',#3253,#3254,#1720,.F.) ;
#3971=EDGE_CURVE('',#3254,#3249,#2717,.F.) ;
#3972=EDGE_CURVE('',#3251,#3255,#1721,.T.) ;
#3973=EDGE_CURVE('',#3255,#3256,#1722,.F.) ;
#3974=EDGE_CURVE('',#3256,#3252,#1723,.T.) ;
#3975=EDGE_CURVE('',#3257,#3258,#2718,.T.) ;
#3976=EDGE_CURVE('',#3257,#3259,#1724,.T.) ;
#3977=EDGE_CURVE('',#3260,#3259,#2719,.T.) ;
#3978=EDGE_CURVE('',#3261,#3260,#1725,.T.) ;
#3979=EDGE_CURVE('',#3262,#3261,#2720,.T.) ;
#3980=EDGE_CURVE('',#3262,#3253,#1726,.T.) ;
#3981=EDGE_CURVE('',#3263,#3256,#2721,.T.) ;
#3982=EDGE_CURVE('',#3263,#3264,#1727,.T.) ;
#3983=EDGE_CURVE('',#3265,#3264,#2722,.T.) ;
#3984=EDGE_CURVE('',#3266,#3265,#1728,.T.) ;
#3985=EDGE_CURVE('',#3267,#3266,#2723,.T.) ;
#3986=EDGE_CURVE('',#3267,#3268,#1729,.T.) ;
#3987=EDGE_CURVE('',#3269,#3268,#2724,.T.) ;
#3988=EDGE_CURVE('',#3270,#3269,#1730,.T.) ;
#3989=EDGE_CURVE('',#3271,#3270,#2725,.T.) ;
#3990=EDGE_CURVE('',#3271,#3272,#1731,.T.) ;
#3991=EDGE_CURVE('',#3273,#3272,#2726,.T.) ;
#3992=EDGE_CURVE('',#3274,#3273,#1732,.T.) ;
#3993=EDGE_CURVE('',#3275,#3274,#2727,.T.) ;
#3994=EDGE_CURVE('',#3275,#3276,#1733,.T.) ;
#3995=EDGE_CURVE('',#3277,#3276,#2728,.T.) ;
#3996=EDGE_CURVE('',#3278,#3277,#1734,.T.) ;
#3997=EDGE_CURVE('',#3279,#3278,#2729,.T.) ;
#3998=EDGE_CURVE('',#3279,#3280,#1735,.T.) ;
#3999=EDGE_CURVE('',#3281,#3280,#2730,.T.) ;
#4000=EDGE_CURVE('',#3282,#3281,#1736,.T.) ;
#4001=EDGE_CURVE('',#3283,#3282,#2731,.T.) ;
#4002=EDGE_CURVE('',#3283,#3284,#1737,.T.) ;
#4003=EDGE_CURVE('',#3285,#3284,#2732,.T.) ;
#4004=EDGE_CURVE('',#3286,#3285,#1738,.T.) ;
#4005=EDGE_CURVE('',#3258,#3286,#2733,.T.) ;
#4006=EDGE_CURVE('',#3258,#3287,#1739,.T.) ;
#4007=EDGE_CURVE('',#3287,#3287,#2734,.T.) ;
#4008=EDGE_CURVE('',#3254,#3288,#1740,.T.) ;
#4009=EDGE_CURVE('',#3262,#3288,#1741,.F.) ;
#4010=EDGE_CURVE('',#3289,#3290,#2735,.T.) ;
#4011=EDGE_CURVE('',#3289,#3291,#2736,.T.) ;
#4012=EDGE_CURVE('',#3263,#3291,#1742,.F.) ;
#4013=EDGE_CURVE('',#3255,#3290,#2737,.T.) ;
#4014=EDGE_CURVE('',#3292,#3291,#1743,.T.) ;
#4015=EDGE_CURVE('',#3264,#3292,#1744,.F.) ;
#4016=EDGE_CURVE('',#3293,#3294,#1745,.T.) ;
#4017=EDGE_CURVE('',#3268,#3293,#1746,.F.) ;
#4018=EDGE_CURVE('',#3267,#3294,#1747,.F.) ;
#4019=EDGE_CURVE('',#3295,#3296,#1748,.F.) ;
#4020=EDGE_CURVE('',#3296,#3297,#2738,.T.) ;
#4021=EDGE_CURVE('',#3297,#3298,#1749,.T.) ;
#4022=EDGE_CURVE('',#3298,#3295,#2739,.T.) ;
#4023=EDGE_CURVE('',#3299,#3300,#1750,.T.) ;
#4024=EDGE_CURVE('',#3259,#3299,#1751,.F.) ;
#4025=EDGE_CURVE('',#3257,#3300,#1752,.F.) ;
#4026=EDGE_CURVE('',#3301,#3302,#2740,.F.) ;
#4027=EDGE_CURVE('',#3302,#3303,#1753,.F.) ;
#4028=EDGE_CURVE('',#3292,#3303,#2741,.T.) ;
#4029=EDGE_CURVE('',#3301,#3289,#1754,.T.) ;
#4030=EDGE_CURVE('',#3304,#3305,#1755,.T.) ;
#4031=EDGE_CURVE('',#3272,#3304,#1756,.F.) ;
#4032=EDGE_CURVE('',#3271,#3305,#1757,.F.) ;
#4033=EDGE_CURVE('',#3306,#3307,#1758,.T.) ;
#4034=EDGE_CURVE('',#3276,#3306,#1759,.F.) ;
#4035=EDGE_CURVE('',#3275,#3307,#1760,.F.) ;
#4036=EDGE_CURVE('',#3308,#3309,#1761,.T.) ;
#4037=EDGE_CURVE('',#3280,#3308,#1762,.F.) ;
#4038=EDGE_CURVE('',#3279,#3309,#1763,.F.) ;
#4039=EDGE_CURVE('',#3310,#3311,#1764,.T.) ;
#4040=EDGE_CURVE('',#3284,#3310,#1765,.F.) ;
#4041=EDGE_CURVE('',#3283,#3311,#1766,.F.) ;
#4042=EDGE_CURVE('',#3312,#3313,#2742,.T.) ;
#4043=EDGE_CURVE('',#3313,#3295,#1767,.F.) ;
#4044=EDGE_CURVE('',#3312,#3298,#1768,.F.) ;
#4045=EDGE_CURVE('',#3314,#3312,#1769,.T.) ;
#4046=EDGE_CURVE('',#3297,#3314,#1770,.T.) ;
#4047=EDGE_CURVE('',#3315,#3314,#2743,.T.) ;
#4048=EDGE_CURVE('',#3315,#3296,#1771,.F.) ;
#4049=EDGE_CURVE('',#3315,#3313,#1772,.T.) ;
#4050=EDGE_CURVE('',#3316,#3303,#2744,.T.) ;
#4051=EDGE_CURVE('',#3317,#3302,#2745,.T.) ;
#4052=EDGE_CURVE('',#3317,#3316,#1773,.T.) ;
#4053=EDGE_CURVE('',#3318,#3319,#1774,.F.) ;
#4054=EDGE_CURVE('',#3318,#3320,#2746,.F.) ;
#4055=EDGE_CURVE('',#3320,#3321,#1775,.T.) ;
#4056=EDGE_CURVE('',#3322,#3321,#2747,.F.) ;
#4057=EDGE_CURVE('',#3323,#3322,#1776,.T.) ;
#4058=EDGE_CURVE('',#3319,#3323,#2748,.T.) ;
#4059=EDGE_CURVE('',#3324,#3325,#2749,.T.) ;
#4060=EDGE_CURVE('',#3326,#3325,#1777,.F.) ;
#4061=EDGE_CURVE('',#3327,#3326,#2750,.T.) ;
#4062=EDGE_CURVE('',#3327,#3324,#1778,.F.) ;
#4063=EDGE_CURVE('',#3328,#3329,#1779,.F.) ;
#4064=EDGE_CURVE('',#3328,#3326,#2751,.F.) ;
#4065=EDGE_CURVE('',#3330,#3325,#2752,.F.) ;
#4066=EDGE_CURVE('',#3331,#3330,#1780,.T.) ;
#4067=EDGE_CURVE('',#3329,#3331,#2753,.T.) ;
#4068=EDGE_CURVE('',#3332,#3333,#2754,.T.) ;
#4069=EDGE_CURVE('',#3332,#3334,#1781,.F.) ;
#4070=EDGE_CURVE('',#3334,#3335,#2755,.T.) ;
#4071=EDGE_CURVE('',#3333,#3335,#1782,.F.) ;
#4072=EDGE_CURVE('',#3336,#3337,#1783,.F.) ;
#4073=EDGE_CURVE('',#3336,#3333,#2756,.F.) ;
#4074=EDGE_CURVE('',#3338,#3335,#2757,.F.) ;
#4075=EDGE_CURVE('',#3339,#3338,#1784,.T.) ;
#4076=EDGE_CURVE('',#3337,#3339,#2758,.T.) ;
#4077=EDGE_CURVE('',#3340,#3341,#2759,.T.) ;
#4078=EDGE_CURVE('',#3340,#3342,#1785,.F.) ;
#4079=EDGE_CURVE('',#3342,#3343,#2760,.T.) ;
#4080=EDGE_CURVE('',#3341,#3343,#1786,.F.) ;
#4081=EDGE_CURVE('',#3344,#3345,#1787,.F.) ;
#4082=EDGE_CURVE('',#3344,#3341,#2761,.F.) ;
#4083=EDGE_CURVE('',#3346,#3343,#2762,.F.) ;
#4084=EDGE_CURVE('',#3347,#3346,#1788,.T.) ;
#4085=EDGE_CURVE('',#3345,#3347,#2763,.T.) ;
#4086=EDGE_CURVE('',#3348,#3349,#2764,.T.) ;
#4087=EDGE_CURVE('',#3348,#3350,#1789,.F.) ;
#4088=EDGE_CURVE('',#3350,#3351,#2765,.T.) ;
#4089=EDGE_CURVE('',#3349,#3351,#1790,.F.) ;
#4090=EDGE_CURVE('',#3352,#3353,#1791,.F.) ;
#4091=EDGE_CURVE('',#3352,#3349,#2766,.F.) ;
#4092=EDGE_CURVE('',#3354,#3351,#2767,.F.) ;
#4093=EDGE_CURVE('',#3355,#3354,#1792,.T.) ;
#4094=EDGE_CURVE('',#3353,#3355,#2768,.T.) ;
#4095=EDGE_CURVE('',#3356,#3357,#2769,.T.) ;
#4096=EDGE_CURVE('',#3358,#3357,#1793,.F.) ;
#4097=EDGE_CURVE('',#3359,#3358,#2770,.T.) ;
#4098=EDGE_CURVE('',#3359,#3356,#1794,.F.) ;
#4099=EDGE_CURVE('',#3360,#3361,#1795,.F.) ;
#4100=EDGE_CURVE('',#3360,#3358,#2771,.F.) ;
#4101=EDGE_CURVE('',#3362,#3357,#2772,.F.) ;
#4102=EDGE_CURVE('',#3363,#3362,#1796,.T.) ;
#4103=EDGE_CURVE('',#3361,#3363,#2773,.T.) ;
#4104=EDGE_CURVE('',#3364,#3365,#2774,.T.) ;
#4105=EDGE_CURVE('',#3364,#3366,#1797,.F.) ;
#4106=EDGE_CURVE('',#3366,#3367,#2775,.T.) ;
#4107=EDGE_CURVE('',#3365,#3367,#1798,.F.) ;
#4108=EDGE_CURVE('',#3337,#3368,#2776,.T.) ;
#4109=EDGE_CURVE('',#3368,#3369,#1799,.F.) ;
#4110=EDGE_CURVE('',#3336,#3369,#2777,.T.) ;
#4111=EDGE_CURVE('',#3361,#3370,#2778,.T.) ;
#4112=EDGE_CURVE('',#3370,#3371,#1800,.F.) ;
#4113=EDGE_CURVE('',#3360,#3371,#2779,.T.) ;
#4114=EDGE_CURVE('',#3353,#3372,#2780,.T.) ;
#4115=EDGE_CURVE('',#3373,#3372,#1801,.T.) ;
#4116=EDGE_CURVE('',#3352,#3373,#2781,.T.) ;
#4117=EDGE_CURVE('',#3345,#3374,#2782,.T.) ;
#4118=EDGE_CURVE('',#3375,#3374,#1802,.T.) ;
#4119=EDGE_CURVE('',#3344,#3375,#2783,.T.) ;
#4120=EDGE_CURVE('',#3329,#3376,#2784,.T.) ;
#4121=EDGE_CURVE('',#3377,#3376,#1803,.T.) ;
#4122=EDGE_CURVE('',#3328,#3377,#2785,.T.) ;
#4123=EDGE_CURVE('',#3319,#3378,#2786,.T.) ;
#4124=EDGE_CURVE('',#3379,#3378,#1804,.T.) ;
#4125=EDGE_CURVE('',#3318,#3379,#2787,.T.) ;
#4126=EDGE_CURVE('',#3380,#3320,#2788,.T.) ;
#4127=EDGE_CURVE('',#3380,#3381,#1805,.F.) ;
#4128=EDGE_CURVE('',#3381,#3321,#2789,.T.) ;
#4129=EDGE_CURVE('',#3317,#3365,#2790,.F.) ;
#4130=EDGE_CURVE('',#3382,#3367,#2791,.F.) ;
#4131=EDGE_CURVE('',#3383,#3382,#1806,.T.) ;
#4132=EDGE_CURVE('',#3316,#3383,#2792,.T.) ;
#4133=EDGE_CURVE('',#3332,#3377,#2793,.F.) ;
#4134=EDGE_CURVE('',#3310,#3376,#2794,.T.) ;
#4135=EDGE_CURVE('',#3334,#3311,#2795,.F.) ;
#4136=EDGE_CURVE('',#3340,#3369,#2796,.F.) ;
#4137=EDGE_CURVE('',#3308,#3368,#2797,.T.) ;
#4138=EDGE_CURVE('',#3342,#3309,#2798,.F.) ;
#4139=EDGE_CURVE('',#3348,#3375,#2799,.F.) ;
#4140=EDGE_CURVE('',#3306,#3374,#2800,.T.) ;
#4141=EDGE_CURVE('',#3350,#3307,#2801,.F.) ;
#4142=EDGE_CURVE('',#3359,#3373,#2802,.F.) ;
#4143=EDGE_CURVE('',#3304,#3372,#2803,.T.) ;
#4144=EDGE_CURVE('',#3356,#3305,#2804,.F.) ;
#4145=EDGE_CURVE('',#3327,#3379,#2805,.F.) ;
#4146=EDGE_CURVE('',#3299,#3378,#2806,.T.) ;
#4147=EDGE_CURVE('',#3324,#3300,#2807,.F.) ;
#4148=EDGE_CURVE('',#3330,#3286,#1807,.F.) ;
#4149=EDGE_CURVE('',#3331,#3285,#1808,.F.) ;
#4150=EDGE_CURVE('',#3338,#3282,#1809,.F.) ;
#4151=EDGE_CURVE('',#3339,#3281,#1810,.F.) ;
#4152=EDGE_CURVE('',#3346,#3278,#1811,.F.) ;
#4153=EDGE_CURVE('',#3347,#3277,#1812,.F.) ;
#4154=EDGE_CURVE('',#3354,#3274,#1813,.F.) ;
#4155=EDGE_CURVE('',#3355,#3273,#1814,.F.) ;
#4156=EDGE_CURVE('',#3364,#3371,#2808,.F.) ;
#4157=EDGE_CURVE('',#3293,#3370,#2809,.T.) ;
#4158=EDGE_CURVE('',#3366,#3294,#2810,.F.) ;
#4159=EDGE_CURVE('',#3301,#3384,#2811,.T.) ;
#4160=EDGE_CURVE('',#3384,#3290,#1815,.F.) ;
#4161=EDGE_CURVE('',#3323,#3260,#1816,.F.) ;
#4162=EDGE_CURVE('',#3362,#3270,#1817,.F.) ;
#4163=EDGE_CURVE('',#3363,#3269,#1818,.F.) ;
#4164=EDGE_CURVE('',#3382,#3266,#1819,.F.) ;
#4165=EDGE_CURVE('',#3383,#3265,#1820,.F.) ;
#4166=EDGE_CURVE('',#3381,#3288,#2812,.T.) ;
#4167=EDGE_CURVE('',#3322,#3261,#1821,.F.) ;
#4168=EDGE_CURVE('',#3247,#3384,#2813,.F.) ;
#4169=EDGE_CURVE('',#3380,#3250,#2814,.F.) ;
#5152=ORIENTED_EDGE('',*,*,#3963,.T.) ;
#5153=ORIENTED_EDGE('',*,*,#3964,.T.) ;
#5154=ORIENTED_EDGE('',*,*,#3965,.T.) ;
#5155=ORIENTED_EDGE('',*,*,#3966,.F.) ;
#5156=ORIENTED_EDGE('',*,*,#3967,.T.) ;
#5157=ORIENTED_EDGE('',*,*,#3968,.T.) ;
#5158=ORIENTED_EDGE('',*,*,#3969,.T.) ;
#5159=ORIENTED_EDGE('',*,*,#3970,.T.) ;
#5160=ORIENTED_EDGE('',*,*,#3971,.T.) ;
#5161=ORIENTED_EDGE('',*,*,#3964,.F.) ;
#5162=ORIENTED_EDGE('',*,*,#3972,.T.) ;
#5163=ORIENTED_EDGE('',*,*,#3973,.T.) ;
#5164=ORIENTED_EDGE('',*,*,#3974,.T.) ;
#5165=ORIENTED_EDGE('',*,*,#3968,.F.) ;
#5166=ORIENTED_EDGE('',*,*,#3975,.F.) ;
#5167=ORIENTED_EDGE('',*,*,#3976,.T.) ;
#5168=ORIENTED_EDGE('',*,*,#3977,.F.) ;
#5169=ORIENTED_EDGE('',*,*,#3978,.F.) ;
#5170=ORIENTED_EDGE('',*,*,#3979,.F.) ;
#5171=ORIENTED_EDGE('',*,*,#3980,.T.) ;
#5172=ORIENTED_EDGE('',*,*,#3969,.F.) ;
#5173=ORIENTED_EDGE('',*,*,#3974,.F.) ;
#5174=ORIENTED_EDGE('',*,*,#3981,.F.) ;
#5175=ORIENTED_EDGE('',*,*,#3982,.T.) ;
#5176=ORIENTED_EDGE('',*,*,#3983,.F.) ;
#5177=ORIENTED_EDGE('',*,*,#3984,.F.) ;
#5178=ORIENTED_EDGE('',*,*,#3985,.F.) ;
#5179=ORIENTED_EDGE('',*,*,#3986,.T.) ;
#5180=ORIENTED_EDGE('',*,*,#3987,.F.) ;
#5181=ORIENTED_EDGE('',*,*,#3988,.F.) ;
#5182=ORIENTED_EDGE('',*,*,#3989,.F.) ;
#5183=ORIENTED_EDGE('',*,*,#3990,.T.) ;
#5184=ORIENTED_EDGE('',*,*,#3991,.F.) ;
#5185=ORIENTED_EDGE('',*,*,#3992,.F.) ;
#5186=ORIENTED_EDGE('',*,*,#3993,.F.) ;
#5187=ORIENTED_EDGE('',*,*,#3994,.T.) ;
#5188=ORIENTED_EDGE('',*,*,#3995,.F.) ;
#5189=ORIENTED_EDGE('',*,*,#3996,.F.) ;
#5190=ORIENTED_EDGE('',*,*,#3997,.F.) ;
#5191=ORIENTED_EDGE('',*,*,#3998,.T.) ;
#5192=ORIENTED_EDGE('',*,*,#3999,.F.) ;
#5193=ORIENTED_EDGE('',*,*,#4000,.F.) ;
#5194=ORIENTED_EDGE('',*,*,#4001,.F.) ;
#5195=ORIENTED_EDGE('',*,*,#4002,.T.) ;
#5196=ORIENTED_EDGE('',*,*,#4003,.F.) ;
#5197=ORIENTED_EDGE('',*,*,#4004,.F.) ;
#5198=ORIENTED_EDGE('',*,*,#4005,.F.) ;
#5199=ORIENTED_EDGE('',*,*,#4006,.T.) ;
#5200=ORIENTED_EDGE('',*,*,#4007,.T.) ;
#5201=ORIENTED_EDGE('',*,*,#4006,.F.) ;
#5202=ORIENTED_EDGE('',*,*,#4008,.F.) ;
#5203=ORIENTED_EDGE('',*,*,#3970,.F.) ;
#5204=ORIENTED_EDGE('',*,*,#3980,.F.) ;
#5205=ORIENTED_EDGE('',*,*,#4009,.T.) ;
#5206=ORIENTED_EDGE('',*,*,#4010,.F.) ;
#5207=ORIENTED_EDGE('',*,*,#4011,.T.) ;
#5208=ORIENTED_EDGE('',*,*,#4012,.F.) ;
#5209=ORIENTED_EDGE('',*,*,#3981,.T.) ;
#5210=ORIENTED_EDGE('',*,*,#3973,.F.) ;
#5211=ORIENTED_EDGE('',*,*,#4013,.T.) ;
#5212=ORIENTED_EDGE('',*,*,#4014,.F.) ;
#5213=ORIENTED_EDGE('',*,*,#4015,.F.) ;
#5214=ORIENTED_EDGE('',*,*,#3982,.F.) ;
#5215=ORIENTED_EDGE('',*,*,#4012,.T.) ;
#5216=ORIENTED_EDGE('',*,*,#4016,.F.) ;
#5217=ORIENTED_EDGE('',*,*,#4017,.F.) ;
#5218=ORIENTED_EDGE('',*,*,#3986,.F.) ;
#5219=ORIENTED_EDGE('',*,*,#4018,.T.) ;
#5220=ORIENTED_EDGE('',*,*,#4007,.F.) ;
#5221=ORIENTED_EDGE('',*,*,#4019,.T.) ;
#5222=ORIENTED_EDGE('',*,*,#4020,.T.) ;
#5223=ORIENTED_EDGE('',*,*,#4021,.T.) ;
#5224=ORIENTED_EDGE('',*,*,#4022,.T.) ;
#5225=ORIENTED_EDGE('',*,*,#4023,.F.) ;
#5226=ORIENTED_EDGE('',*,*,#4024,.F.) ;
#5227=ORIENTED_EDGE('',*,*,#3976,.F.) ;
#5228=ORIENTED_EDGE('',*,*,#4025,.T.) ;
#5229=ORIENTED_EDGE('',*,*,#4026,.T.) ;
#5230=ORIENTED_EDGE('',*,*,#4027,.T.) ;
#5231=ORIENTED_EDGE('',*,*,#4028,.F.) ;
#5232=ORIENTED_EDGE('',*,*,#4014,.T.) ;
#5233=ORIENTED_EDGE('',*,*,#4011,.F.) ;
#5234=ORIENTED_EDGE('',*,*,#4029,.F.) ;
#5235=ORIENTED_EDGE('',*,*,#4030,.F.) ;
#5236=ORIENTED_EDGE('',*,*,#4031,.F.) ;
#5237=ORIENTED_EDGE('',*,*,#3990,.F.) ;
#5238=ORIENTED_EDGE('',*,*,#4032,.T.) ;
#5239=ORIENTED_EDGE('',*,*,#4033,.F.) ;
#5240=ORIENTED_EDGE('',*,*,#4034,.F.) ;
#5241=ORIENTED_EDGE('',*,*,#3994,.F.) ;
#5242=ORIENTED_EDGE('',*,*,#4035,.T.) ;
#5243=ORIENTED_EDGE('',*,*,#4036,.F.) ;
#5244=ORIENTED_EDGE('',*,*,#4037,.F.) ;
#5245=ORIENTED_EDGE('',*,*,#3998,.F.) ;
#5246=ORIENTED_EDGE('',*,*,#4038,.T.) ;
#5247=ORIENTED_EDGE('',*,*,#4039,.F.) ;
#5248=ORIENTED_EDGE('',*,*,#4040,.F.) ;
#5249=ORIENTED_EDGE('',*,*,#4002,.F.) ;
#5250=ORIENTED_EDGE('',*,*,#4041,.T.) ;
#5251=ORIENTED_EDGE('',*,*,#4042,.T.) ;
#5252=ORIENTED_EDGE('',*,*,#4043,.T.) ;
#5253=ORIENTED_EDGE('',*,*,#4022,.F.) ;
#5254=ORIENTED_EDGE('',*,*,#4044,.F.) ;
#5255=ORIENTED_EDGE('',*,*,#4045,.T.) ;
#5256=ORIENTED_EDGE('',*,*,#4044,.T.) ;
#5257=ORIENTED_EDGE('',*,*,#4021,.F.) ;
#5258=ORIENTED_EDGE('',*,*,#4046,.T.) ;
#5259=ORIENTED_EDGE('',*,*,#4047,.T.) ;
#5260=ORIENTED_EDGE('',*,*,#4046,.F.) ;
#5261=ORIENTED_EDGE('',*,*,#4020,.F.) ;
#5262=ORIENTED_EDGE('',*,*,#4048,.F.) ;
#5263=ORIENTED_EDGE('',*,*,#4048,.T.) ;
#5264=ORIENTED_EDGE('',*,*,#4019,.F.) ;
#5265=ORIENTED_EDGE('',*,*,#4043,.F.) ;
#5266=ORIENTED_EDGE('',*,*,#4049,.F.) ;
#5267=ORIENTED_EDGE('',*,*,#4050,.T.) ;
#5268=ORIENTED_EDGE('',*,*,#4027,.F.) ;
#5269=ORIENTED_EDGE('',*,*,#4051,.F.) ;
#5270=ORIENTED_EDGE('',*,*,#4052,.T.) ;
#5271=ORIENTED_EDGE('',*,*,#4053,.F.) ;
#5272=ORIENTED_EDGE('',*,*,#4054,.T.) ;
#5273=ORIENTED_EDGE('',*,*,#4055,.T.) ;
#5274=ORIENTED_EDGE('',*,*,#4056,.F.) ;
#5275=ORIENTED_EDGE('',*,*,#4057,.F.) ;
#5276=ORIENTED_EDGE('',*,*,#4058,.F.) ;
#5277=ORIENTED_EDGE('',*,*,#4059,.T.) ;
#5278=ORIENTED_EDGE('',*,*,#4060,.F.) ;
#5279=ORIENTED_EDGE('',*,*,#4061,.F.) ;
#5280=ORIENTED_EDGE('',*,*,#4062,.T.) ;
#5281=ORIENTED_EDGE('',*,*,#4063,.F.) ;
#5282=ORIENTED_EDGE('',*,*,#4064,.T.) ;
#5283=ORIENTED_EDGE('',*,*,#4060,.T.) ;
#5284=ORIENTED_EDGE('',*,*,#4065,.F.) ;
#5285=ORIENTED_EDGE('',*,*,#4066,.F.) ;
#5286=ORIENTED_EDGE('',*,*,#4067,.F.) ;
#5287=ORIENTED_EDGE('',*,*,#4068,.F.) ;
#5288=ORIENTED_EDGE('',*,*,#4069,.T.) ;
#5289=ORIENTED_EDGE('',*,*,#4070,.T.) ;
#5290=ORIENTED_EDGE('',*,*,#4071,.F.) ;
#5291=ORIENTED_EDGE('',*,*,#4072,.F.) ;
#5292=ORIENTED_EDGE('',*,*,#4073,.T.) ;
#5293=ORIENTED_EDGE('',*,*,#4071,.T.) ;
#5294=ORIENTED_EDGE('',*,*,#4074,.F.) ;
#5295=ORIENTED_EDGE('',*,*,#4075,.F.) ;
#5296=ORIENTED_EDGE('',*,*,#4076,.F.) ;
#5297=ORIENTED_EDGE('',*,*,#4077,.F.) ;
#5298=ORIENTED_EDGE('',*,*,#4078,.T.) ;
#5299=ORIENTED_EDGE('',*,*,#4079,.T.) ;
#5300=ORIENTED_EDGE('',*,*,#4080,.F.) ;
#5301=ORIENTED_EDGE('',*,*,#4081,.F.) ;
#5302=ORIENTED_EDGE('',*,*,#4082,.T.) ;
#5303=ORIENTED_EDGE('',*,*,#4080,.T.) ;
#5304=ORIENTED_EDGE('',*,*,#4083,.F.) ;
#5305=ORIENTED_EDGE('',*,*,#4084,.F.) ;
#5306=ORIENTED_EDGE('',*,*,#4085,.F.) ;
#5307=ORIENTED_EDGE('',*,*,#4086,.F.) ;
#5308=ORIENTED_EDGE('',*,*,#4087,.T.) ;
#5309=ORIENTED_EDGE('',*,*,#4088,.T.) ;
#5310=ORIENTED_EDGE('',*,*,#4089,.F.) ;
#5311=ORIENTED_EDGE('',*,*,#4090,.F.) ;
#5312=ORIENTED_EDGE('',*,*,#4091,.T.) ;
#5313=ORIENTED_EDGE('',*,*,#4089,.T.) ;
#5314=ORIENTED_EDGE('',*,*,#4092,.F.) ;
#5315=ORIENTED_EDGE('',*,*,#4093,.F.) ;
#5316=ORIENTED_EDGE('',*,*,#4094,.F.) ;
#5317=ORIENTED_EDGE('',*,*,#4095,.T.) ;
#5318=ORIENTED_EDGE('',*,*,#4096,.F.) ;
#5319=ORIENTED_EDGE('',*,*,#4097,.F.) ;
#5320=ORIENTED_EDGE('',*,*,#4098,.T.) ;
#5321=ORIENTED_EDGE('',*,*,#4099,.F.) ;
#5322=ORIENTED_EDGE('',*,*,#4100,.T.) ;
#5323=ORIENTED_EDGE('',*,*,#4096,.T.) ;
#5324=ORIENTED_EDGE('',*,*,#4101,.F.) ;
#5325=ORIENTED_EDGE('',*,*,#4102,.F.) ;
#5326=ORIENTED_EDGE('',*,*,#4103,.F.) ;
#5327=ORIENTED_EDGE('',*,*,#4104,.F.) ;
#5328=ORIENTED_EDGE('',*,*,#4105,.T.) ;
#5329=ORIENTED_EDGE('',*,*,#4106,.T.) ;
#5330=ORIENTED_EDGE('',*,*,#4107,.F.) ;
#5331=ORIENTED_EDGE('',*,*,#4108,.T.) ;
#5332=ORIENTED_EDGE('',*,*,#4109,.T.) ;
#5333=ORIENTED_EDGE('',*,*,#4110,.F.) ;
#5334=ORIENTED_EDGE('',*,*,#4072,.T.) ;
#5335=ORIENTED_EDGE('',*,*,#4099,.T.) ;
#5336=ORIENTED_EDGE('',*,*,#4111,.T.) ;
#5337=ORIENTED_EDGE('',*,*,#4112,.T.) ;
#5338=ORIENTED_EDGE('',*,*,#4113,.F.) ;
#5339=ORIENTED_EDGE('',*,*,#4090,.T.) ;
#5340=ORIENTED_EDGE('',*,*,#4114,.T.) ;
#5341=ORIENTED_EDGE('',*,*,#4115,.F.) ;
#5342=ORIENTED_EDGE('',*,*,#4116,.F.) ;
#5343=ORIENTED_EDGE('',*,*,#4081,.T.) ;
#5344=ORIENTED_EDGE('',*,*,#4117,.T.) ;
#5345=ORIENTED_EDGE('',*,*,#4118,.F.) ;
#5346=ORIENTED_EDGE('',*,*,#4119,.F.) ;
#5347=ORIENTED_EDGE('',*,*,#4063,.T.) ;
#5348=ORIENTED_EDGE('',*,*,#4120,.T.) ;
#5349=ORIENTED_EDGE('',*,*,#4121,.F.) ;
#5350=ORIENTED_EDGE('',*,*,#4122,.F.) ;
#5351=ORIENTED_EDGE('',*,*,#4053,.T.) ;
#5352=ORIENTED_EDGE('',*,*,#4123,.T.) ;
#5353=ORIENTED_EDGE('',*,*,#4124,.F.) ;
#5354=ORIENTED_EDGE('',*,*,#4125,.F.) ;
#5355=ORIENTED_EDGE('',*,*,#4126,.F.) ;
#5356=ORIENTED_EDGE('',*,*,#4127,.T.) ;
#5357=ORIENTED_EDGE('',*,*,#4128,.T.) ;
#5358=ORIENTED_EDGE('',*,*,#4055,.F.) ;
#5359=ORIENTED_EDGE('',*,*,#4052,.F.) ;
#5360=ORIENTED_EDGE('',*,*,#4129,.T.) ;
#5361=ORIENTED_EDGE('',*,*,#4107,.T.) ;
#5362=ORIENTED_EDGE('',*,*,#4130,.F.) ;
#5363=ORIENTED_EDGE('',*,*,#4131,.F.) ;
#5364=ORIENTED_EDGE('',*,*,#4132,.F.) ;
#5365=ORIENTED_EDGE('',*,*,#4133,.T.) ;
#5366=ORIENTED_EDGE('',*,*,#4121,.T.) ;
#5367=ORIENTED_EDGE('',*,*,#4134,.F.) ;
#5368=ORIENTED_EDGE('',*,*,#4039,.T.) ;
#5369=ORIENTED_EDGE('',*,*,#4135,.F.) ;
#5370=ORIENTED_EDGE('',*,*,#4069,.F.) ;
#5371=ORIENTED_EDGE('',*,*,#4136,.T.) ;
#5372=ORIENTED_EDGE('',*,*,#4109,.F.) ;
#5373=ORIENTED_EDGE('',*,*,#4137,.F.) ;
#5374=ORIENTED_EDGE('',*,*,#4036,.T.) ;
#5375=ORIENTED_EDGE('',*,*,#4138,.F.) ;
#5376=ORIENTED_EDGE('',*,*,#4078,.F.) ;
#5377=ORIENTED_EDGE('',*,*,#4139,.T.) ;
#5378=ORIENTED_EDGE('',*,*,#4118,.T.) ;
#5379=ORIENTED_EDGE('',*,*,#4140,.F.) ;
#5380=ORIENTED_EDGE('',*,*,#4033,.T.) ;
#5381=ORIENTED_EDGE('',*,*,#4141,.F.) ;
#5382=ORIENTED_EDGE('',*,*,#4087,.F.) ;
#5383=ORIENTED_EDGE('',*,*,#4142,.T.) ;
#5384=ORIENTED_EDGE('',*,*,#4115,.T.) ;
#5385=ORIENTED_EDGE('',*,*,#4143,.F.) ;
#5386=ORIENTED_EDGE('',*,*,#4030,.T.) ;
#5387=ORIENTED_EDGE('',*,*,#4144,.F.) ;
#5388=ORIENTED_EDGE('',*,*,#4098,.F.) ;
#5389=ORIENTED_EDGE('',*,*,#4145,.T.) ;
#5390=ORIENTED_EDGE('',*,*,#4124,.T.) ;
#5391=ORIENTED_EDGE('',*,*,#4146,.F.) ;
#5392=ORIENTED_EDGE('',*,*,#4023,.T.) ;
#5393=ORIENTED_EDGE('',*,*,#4147,.F.) ;
#5394=ORIENTED_EDGE('',*,*,#4062,.F.) ;
#5395=ORIENTED_EDGE('',*,*,#4066,.T.) ;
#5396=ORIENTED_EDGE('',*,*,#4148,.T.) ;
#5397=ORIENTED_EDGE('',*,*,#4004,.T.) ;
#5398=ORIENTED_EDGE('',*,*,#4149,.F.) ;
#5399=ORIENTED_EDGE('',*,*,#4067,.T.) ;
#5400=ORIENTED_EDGE('',*,*,#4149,.T.) ;
#5401=ORIENTED_EDGE('',*,*,#4003,.T.) ;
#5402=ORIENTED_EDGE('',*,*,#4040,.T.) ;
#5403=ORIENTED_EDGE('',*,*,#4134,.T.) ;
#5404=ORIENTED_EDGE('',*,*,#4120,.F.) ;
#5405=ORIENTED_EDGE('',*,*,#4070,.F.) ;
#5406=ORIENTED_EDGE('',*,*,#4135,.T.) ;
#5407=ORIENTED_EDGE('',*,*,#4041,.F.) ;
#5408=ORIENTED_EDGE('',*,*,#4001,.T.) ;
#5409=ORIENTED_EDGE('',*,*,#4150,.F.) ;
#5410=ORIENTED_EDGE('',*,*,#4074,.T.) ;
#5411=ORIENTED_EDGE('',*,*,#4075,.T.) ;
#5412=ORIENTED_EDGE('',*,*,#4150,.T.) ;
#5413=ORIENTED_EDGE('',*,*,#4000,.T.) ;
#5414=ORIENTED_EDGE('',*,*,#4151,.F.) ;
#5415=ORIENTED_EDGE('',*,*,#4076,.T.) ;
#5416=ORIENTED_EDGE('',*,*,#4151,.T.) ;
#5417=ORIENTED_EDGE('',*,*,#3999,.T.) ;
#5418=ORIENTED_EDGE('',*,*,#4037,.T.) ;
#5419=ORIENTED_EDGE('',*,*,#4137,.T.) ;
#5420=ORIENTED_EDGE('',*,*,#4108,.F.) ;
#5421=ORIENTED_EDGE('',*,*,#4079,.F.) ;
#5422=ORIENTED_EDGE('',*,*,#4138,.T.) ;
#5423=ORIENTED_EDGE('',*,*,#4038,.F.) ;
#5424=ORIENTED_EDGE('',*,*,#3997,.T.) ;
#5425=ORIENTED_EDGE('',*,*,#4152,.F.) ;
#5426=ORIENTED_EDGE('',*,*,#4083,.T.) ;
#5427=ORIENTED_EDGE('',*,*,#4084,.T.) ;
#5428=ORIENTED_EDGE('',*,*,#4152,.T.) ;
#5429=ORIENTED_EDGE('',*,*,#3996,.T.) ;
#5430=ORIENTED_EDGE('',*,*,#4153,.F.) ;
#5431=ORIENTED_EDGE('',*,*,#4085,.T.) ;
#5432=ORIENTED_EDGE('',*,*,#4153,.T.) ;
#5433=ORIENTED_EDGE('',*,*,#3995,.T.) ;
#5434=ORIENTED_EDGE('',*,*,#4034,.T.) ;
#5435=ORIENTED_EDGE('',*,*,#4140,.T.) ;
#5436=ORIENTED_EDGE('',*,*,#4117,.F.) ;
#5437=ORIENTED_EDGE('',*,*,#4088,.F.) ;
#5438=ORIENTED_EDGE('',*,*,#4141,.T.) ;
#5439=ORIENTED_EDGE('',*,*,#4035,.F.) ;
#5440=ORIENTED_EDGE('',*,*,#3993,.T.) ;
#5441=ORIENTED_EDGE('',*,*,#4154,.F.) ;
#5442=ORIENTED_EDGE('',*,*,#4092,.T.) ;
#5443=ORIENTED_EDGE('',*,*,#4093,.T.) ;
#5444=ORIENTED_EDGE('',*,*,#4154,.T.) ;
#5445=ORIENTED_EDGE('',*,*,#3992,.T.) ;
#5446=ORIENTED_EDGE('',*,*,#4155,.F.) ;
#5447=ORIENTED_EDGE('',*,*,#4094,.T.) ;
#5448=ORIENTED_EDGE('',*,*,#4155,.T.) ;
#5449=ORIENTED_EDGE('',*,*,#3991,.T.) ;
#5450=ORIENTED_EDGE('',*,*,#4031,.T.) ;
#5451=ORIENTED_EDGE('',*,*,#4143,.T.) ;
#5452=ORIENTED_EDGE('',*,*,#4114,.F.) ;
#5453=ORIENTED_EDGE('',*,*,#4156,.T.) ;
#5454=ORIENTED_EDGE('',*,*,#4112,.F.) ;
#5455=ORIENTED_EDGE('',*,*,#4157,.F.) ;
#5456=ORIENTED_EDGE('',*,*,#4016,.T.) ;
#5457=ORIENTED_EDGE('',*,*,#4158,.F.) ;
#5458=ORIENTED_EDGE('',*,*,#4105,.F.) ;
#5459=ORIENTED_EDGE('',*,*,#4159,.F.) ;
#5460=ORIENTED_EDGE('',*,*,#4029,.T.) ;
#5461=ORIENTED_EDGE('',*,*,#4010,.T.) ;
#5462=ORIENTED_EDGE('',*,*,#4160,.F.) ;
#5463=ORIENTED_EDGE('',*,*,#4123,.F.) ;
#5464=ORIENTED_EDGE('',*,*,#4058,.T.) ;
#5465=ORIENTED_EDGE('',*,*,#4161,.T.) ;
#5466=ORIENTED_EDGE('',*,*,#3977,.T.) ;
#5467=ORIENTED_EDGE('',*,*,#4024,.T.) ;
#5468=ORIENTED_EDGE('',*,*,#4146,.T.) ;
#5469=ORIENTED_EDGE('',*,*,#4059,.F.) ;
#5470=ORIENTED_EDGE('',*,*,#4147,.T.) ;
#5471=ORIENTED_EDGE('',*,*,#4025,.F.) ;
#5472=ORIENTED_EDGE('',*,*,#3975,.T.) ;
#5473=ORIENTED_EDGE('',*,*,#4005,.T.) ;
#5474=ORIENTED_EDGE('',*,*,#4148,.F.) ;
#5475=ORIENTED_EDGE('',*,*,#4065,.T.) ;
#5476=ORIENTED_EDGE('',*,*,#4095,.F.) ;
#5477=ORIENTED_EDGE('',*,*,#4144,.T.) ;
#5478=ORIENTED_EDGE('',*,*,#4032,.F.) ;
#5479=ORIENTED_EDGE('',*,*,#3989,.T.) ;
#5480=ORIENTED_EDGE('',*,*,#4162,.F.) ;
#5481=ORIENTED_EDGE('',*,*,#4101,.T.) ;
#5482=ORIENTED_EDGE('',*,*,#4102,.T.) ;
#5483=ORIENTED_EDGE('',*,*,#4162,.T.) ;
#5484=ORIENTED_EDGE('',*,*,#3988,.T.) ;
#5485=ORIENTED_EDGE('',*,*,#4163,.F.) ;
#5486=ORIENTED_EDGE('',*,*,#4103,.T.) ;
#5487=ORIENTED_EDGE('',*,*,#4163,.T.) ;
#5488=ORIENTED_EDGE('',*,*,#3987,.T.) ;
#5489=ORIENTED_EDGE('',*,*,#4017,.T.) ;
#5490=ORIENTED_EDGE('',*,*,#4157,.T.) ;
#5491=ORIENTED_EDGE('',*,*,#4111,.F.) ;
#5492=ORIENTED_EDGE('',*,*,#4106,.F.) ;
#5493=ORIENTED_EDGE('',*,*,#4158,.T.) ;
#5494=ORIENTED_EDGE('',*,*,#4018,.F.) ;
#5495=ORIENTED_EDGE('',*,*,#3985,.T.) ;
#5496=ORIENTED_EDGE('',*,*,#4164,.F.) ;
#5497=ORIENTED_EDGE('',*,*,#4130,.T.) ;
#5498=ORIENTED_EDGE('',*,*,#4131,.T.) ;
#5499=ORIENTED_EDGE('',*,*,#4164,.T.) ;
#5500=ORIENTED_EDGE('',*,*,#3984,.T.) ;
#5501=ORIENTED_EDGE('',*,*,#4165,.F.) ;
#5502=ORIENTED_EDGE('',*,*,#4132,.T.) ;
#5503=ORIENTED_EDGE('',*,*,#4165,.T.) ;
#5504=ORIENTED_EDGE('',*,*,#3983,.T.) ;
#5505=ORIENTED_EDGE('',*,*,#4015,.T.) ;
#5506=ORIENTED_EDGE('',*,*,#4028,.T.) ;
#5507=ORIENTED_EDGE('',*,*,#4050,.F.) ;
#5508=ORIENTED_EDGE('',*,*,#4128,.F.) ;
#5509=ORIENTED_EDGE('',*,*,#4166,.T.) ;
#5510=ORIENTED_EDGE('',*,*,#4009,.F.) ;
#5511=ORIENTED_EDGE('',*,*,#3979,.T.) ;
#5512=ORIENTED_EDGE('',*,*,#4167,.F.) ;
#5513=ORIENTED_EDGE('',*,*,#4056,.T.) ;
#5514=ORIENTED_EDGE('',*,*,#4057,.T.) ;
#5515=ORIENTED_EDGE('',*,*,#4167,.T.) ;
#5516=ORIENTED_EDGE('',*,*,#3978,.T.) ;
#5517=ORIENTED_EDGE('',*,*,#4161,.F.) ;
#5518=ORIENTED_EDGE('',*,*,#3963,.F.) ;
#5519=ORIENTED_EDGE('',*,*,#4168,.T.) ;
#5520=ORIENTED_EDGE('',*,*,#4160,.T.) ;
#5521=ORIENTED_EDGE('',*,*,#4013,.F.) ;
#5522=ORIENTED_EDGE('',*,*,#3972,.F.) ;
#5523=ORIENTED_EDGE('',*,*,#3967,.F.) ;
#5524=ORIENTED_EDGE('',*,*,#4169,.T.) ;
#5525=ORIENTED_EDGE('',*,*,#3965,.F.) ;
#5526=ORIENTED_EDGE('',*,*,#3971,.F.) ;
#5527=ORIENTED_EDGE('',*,*,#4008,.T.) ;
#5528=ORIENTED_EDGE('',*,*,#4166,.F.) ;
#5529=ORIENTED_EDGE('',*,*,#4127,.F.) ;
#5530=ORIENTED_EDGE('',*,*,#4129,.F.) ;
#5531=ORIENTED_EDGE('',*,*,#4051,.T.) ;
#5532=ORIENTED_EDGE('',*,*,#4026,.F.) ;
#5533=ORIENTED_EDGE('',*,*,#4159,.T.) ;
#5534=ORIENTED_EDGE('',*,*,#4168,.F.) ;
#5535=ORIENTED_EDGE('',*,*,#3966,.T.) ;
#5536=ORIENTED_EDGE('',*,*,#4169,.F.) ;
#5537=ORIENTED_EDGE('',*,*,#4126,.T.) ;
#5538=ORIENTED_EDGE('',*,*,#4054,.F.) ;
#5539=ORIENTED_EDGE('',*,*,#4125,.T.) ;
#5540=ORIENTED_EDGE('',*,*,#4145,.F.) ;
#5541=ORIENTED_EDGE('',*,*,#4061,.T.) ;
#5542=ORIENTED_EDGE('',*,*,#4064,.F.) ;
#5543=ORIENTED_EDGE('',*,*,#4122,.T.) ;
#5544=ORIENTED_EDGE('',*,*,#4133,.F.) ;
#5545=ORIENTED_EDGE('',*,*,#4068,.T.) ;
#5546=ORIENTED_EDGE('',*,*,#4073,.F.) ;
#5547=ORIENTED_EDGE('',*,*,#4110,.T.) ;
#5548=ORIENTED_EDGE('',*,*,#4136,.F.) ;
#5549=ORIENTED_EDGE('',*,*,#4077,.T.) ;
#5550=ORIENTED_EDGE('',*,*,#4082,.F.) ;
#5551=ORIENTED_EDGE('',*,*,#4119,.T.) ;
#5552=ORIENTED_EDGE('',*,*,#4139,.F.) ;
#5553=ORIENTED_EDGE('',*,*,#4086,.T.) ;
#5554=ORIENTED_EDGE('',*,*,#4091,.F.) ;
#5555=ORIENTED_EDGE('',*,*,#4116,.T.) ;
#5556=ORIENTED_EDGE('',*,*,#4142,.F.) ;
#5557=ORIENTED_EDGE('',*,*,#4097,.T.) ;
#5558=ORIENTED_EDGE('',*,*,#4100,.F.) ;
#5559=ORIENTED_EDGE('',*,*,#4113,.T.) ;
#5560=ORIENTED_EDGE('',*,*,#4156,.F.) ;
#5561=ORIENTED_EDGE('',*,*,#4104,.T.) ;
#5562=ORIENTED_EDGE('',*,*,#4045,.F.) ;
#5563=ORIENTED_EDGE('',*,*,#4047,.F.) ;
#5564=ORIENTED_EDGE('',*,*,#4049,.T.) ;
#5565=ORIENTED_EDGE('',*,*,#4042,.F.) ;
#6983=ADVANCED_FACE('',(#733),#566,.F.) ;
#6984=ADVANCED_FACE('',(#734),#288,.T.) ;
#6985=ADVANCED_FACE('',(#735),#289,.F.) ;
#6986=ADVANCED_FACE('',(#736),#567,.T.) ;
#6987=ADVANCED_FACE('',(#737),#290,.F.) ;
#6988=ADVANCED_FACE('',(#738),#291,.T.) ;
#6989=ADVANCED_FACE('',(#739),#292,.F.) ;
#6990=ADVANCED_FACE('',(#740),#293,.F.) ;
#6991=ADVANCED_FACE('',(#741,#215),#294,.F.) ;
#6992=ADVANCED_FACE('',(#742),#295,.F.) ;
#6993=ADVANCED_FACE('',(#743),#568,.F.) ;
#6994=ADVANCED_FACE('',(#744),#296,.F.) ;
#6995=ADVANCED_FACE('',(#745),#297,.F.) ;
#6996=ADVANCED_FACE('',(#746),#298,.F.) ;
#6997=ADVANCED_FACE('',(#747),#299,.F.) ;
#6998=ADVANCED_FACE('',(#748),#569,.F.) ;
#6999=ADVANCED_FACE('',(#749),#300,.F.) ;
#7000=ADVANCED_FACE('',(#750),#570,.F.) ;
#7001=ADVANCED_FACE('',(#751),#301,.T.) ;
#7002=ADVANCED_FACE('',(#752),#571,.F.) ;
#7003=ADVANCED_FACE('',(#753),#572,.F.) ;
#7004=ADVANCED_FACE('',(#754),#573,.T.) ;
#7005=ADVANCED_FACE('',(#755),#574,.F.) ;
#7006=ADVANCED_FACE('',(#756),#575,.T.) ;
#7007=ADVANCED_FACE('',(#757),#576,.F.) ;
#7008=ADVANCED_FACE('',(#758),#577,.T.) ;
#7009=ADVANCED_FACE('',(#759),#578,.F.) ;
#7010=ADVANCED_FACE('',(#760),#579,.T.) ;
#7011=ADVANCED_FACE('',(#761),#580,.F.) ;
#7012=ADVANCED_FACE('',(#762),#581,.T.) ;
#7013=ADVANCED_FACE('',(#763),#582,.F.) ;
#7014=ADVANCED_FACE('',(#764),#583,.T.) ;
#7015=ADVANCED_FACE('',(#765),#584,.F.) ;
#7016=ADVANCED_FACE('',(#766),#585,.F.) ;
#7017=ADVANCED_FACE('',(#767),#586,.F.) ;
#7018=ADVANCED_FACE('',(#768),#587,.F.) ;
#7019=ADVANCED_FACE('',(#769),#588,.F.) ;
#7020=ADVANCED_FACE('',(#770),#589,.F.) ;
#7021=ADVANCED_FACE('',(#771),#590,.T.) ;
#7022=ADVANCED_FACE('',(#772),#591,.F.) ;
#7023=ADVANCED_FACE('',(#773),#592,.F.) ;
#7024=ADVANCED_FACE('',(#774),#593,.F.) ;
#7025=ADVANCED_FACE('',(#775),#594,.F.) ;
#7026=ADVANCED_FACE('',(#776),#595,.F.) ;
#7027=ADVANCED_FACE('',(#777),#596,.F.) ;
#7028=ADVANCED_FACE('',(#778),#302,.F.) ;
#7029=ADVANCED_FACE('',(#779),#303,.T.) ;
#7030=ADVANCED_FACE('',(#780),#304,.T.) ;
#7031=ADVANCED_FACE('',(#781),#305,.F.) ;
#7032=ADVANCED_FACE('',(#782),#306,.T.) ;
#7033=ADVANCED_FACE('',(#783),#307,.T.) ;
#7034=ADVANCED_FACE('',(#784),#308,.F.) ;
#7035=ADVANCED_FACE('',(#785),#309,.T.) ;
#7036=ADVANCED_FACE('',(#786),#310,.T.) ;
#7037=ADVANCED_FACE('',(#787),#311,.F.) ;
#7038=ADVANCED_FACE('',(#788),#312,.T.) ;
#7039=ADVANCED_FACE('',(#789),#597,.F.) ;
#7040=ADVANCED_FACE('',(#790),#598,.T.) ;
#7041=ADVANCED_FACE('',(#791),#313,.T.) ;
#7042=ADVANCED_FACE('',(#792),#314,.T.) ;
#7043=ADVANCED_FACE('',(#793),#315,.T.) ;
#7044=ADVANCED_FACE('',(#794),#316,.F.) ;
#7045=ADVANCED_FACE('',(#795),#317,.T.) ;
#7046=ADVANCED_FACE('',(#796),#318,.T.) ;
#7047=ADVANCED_FACE('',(#797),#319,.F.) ;
#7048=ADVANCED_FACE('',(#798),#320,.T.) ;
#7049=ADVANCED_FACE('',(#799),#321,.T.) ;
#7050=ADVANCED_FACE('',(#800),#322,.F.) ;
#7051=ADVANCED_FACE('',(#801),#599,.F.) ;
#7052=ADVANCED_FACE('',(#802),#600,.F.) ;
#7053=ADVANCED_FACE('',(#803,#216),#323,.T.) ;
#7373=CLOSED_SHELL('',(#6983,#6984,#6985,#6986,#6987,#6988,#6989,#6990,
#6991,#6992,#6993,#6994,#6995,#6996,#6997,#6998,#6999,#7000,#7001,#7002,
#7003,#7004,#7005,#7006,#7007,#7008,#7009,#7010,#7011,#7012,#7013,#7014,
#7015,#7016,#7017,#7018,#7019,#7020,#7021,#7022,#7023,#7024,#7025,#7026,
#7027,#7028,#7029,#7030,#7031,#7032,#7033,#7034,#7035,#7036,#7037,#7038,
#7039,#7040,#7041,#7042,#7043,#7044,#7045,#7046,#7047,#7048,#7049,#7050,
#7051,#7052,#7053)) ;
#7719=AXIS2_PLACEMENT_3D('',#11550,#8933,#8934) ;
#7720=AXIS2_PLACEMENT_3D('',#11551,#8935,#8936) ;
#7721=AXIS2_PLACEMENT_3D('',#11556,#8938,#8939) ;
#7722=AXIS2_PLACEMENT_3D('',#11559,#8941,#8942) ;
#7723=AXIS2_PLACEMENT_3D('',#11560,#8943,#8944) ;
#7724=AXIS2_PLACEMENT_3D('',#11562,#8945,#8946) ;
#7725=AXIS2_PLACEMENT_3D('',#11566,#8948,#8949) ;
#7726=AXIS2_PLACEMENT_3D('',#11569,#8951,#8952) ;
#7727=AXIS2_PLACEMENT_3D('',#11570,#8953,#8954) ;
#7728=AXIS2_PLACEMENT_3D('',#11576,#8958,#8959) ;
#7729=AXIS2_PLACEMENT_3D('',#11579,#8960,#8961) ;
#7730=AXIS2_PLACEMENT_3D('',#11583,#8963,#8964) ;
#7731=AXIS2_PLACEMENT_3D('',#11587,#8966,#8967) ;
#7732=AXIS2_PLACEMENT_3D('',#11590,#8969,#8970) ;
#7733=AXIS2_PLACEMENT_3D('',#11594,#8972,#8973) ;
#7734=AXIS2_PLACEMENT_3D('',#11598,#8975,#8976) ;
#7735=AXIS2_PLACEMENT_3D('',#11602,#8978,#8979) ;
#7736=AXIS2_PLACEMENT_3D('',#11606,#8981,#8982) ;
#7737=AXIS2_PLACEMENT_3D('',#11610,#8984,#8985) ;
#7738=AXIS2_PLACEMENT_3D('',#11614,#8987,#8988) ;
#7739=AXIS2_PLACEMENT_3D('',#11618,#8990,#8991) ;
#7740=AXIS2_PLACEMENT_3D('',#11622,#8993,#8994) ;
#7741=AXIS2_PLACEMENT_3D('',#11626,#8996,#8997) ;
#7742=AXIS2_PLACEMENT_3D('',#11630,#8999,#9000) ;
#7743=AXIS2_PLACEMENT_3D('',#11634,#9002,#9003) ;
#7744=AXIS2_PLACEMENT_3D('',#11637,#9005,#9006) ;
#7745=AXIS2_PLACEMENT_3D('',#11640,#9008,#9009) ;
#7746=AXIS2_PLACEMENT_3D('',#11641,#9010,#9011) ;
#7747=AXIS2_PLACEMENT_3D('',#11645,#9014,#9015) ;
#7748=AXIS2_PLACEMENT_3D('',#11648,#9016,#9017) ;
#7749=AXIS2_PLACEMENT_3D('',#11650,#9018,#9019) ;
#7750=AXIS2_PLACEMENT_3D('',#11652,#9021,#9022) ;
#7751=AXIS2_PLACEMENT_3D('',#11653,#9023,#9024) ;
#7752=AXIS2_PLACEMENT_3D('',#11657,#9027,#9028) ;
#7753=AXIS2_PLACEMENT_3D('',#11663,#9032,#9033) ;
#7754=AXIS2_PLACEMENT_3D('',#11668,#9035,#9036) ;
#7755=AXIS2_PLACEMENT_3D('',#11671,#9038,#9039) ;
#7756=AXIS2_PLACEMENT_3D('',#11672,#9040,#9041) ;
#7757=AXIS2_PLACEMENT_3D('',#11678,#9045,#9046) ;
#7758=AXIS2_PLACEMENT_3D('',#11681,#9047,#9048) ;
#7759=AXIS2_PLACEMENT_3D('',#11684,#9050,#9051) ;
#7760=AXIS2_PLACEMENT_3D('',#11686,#9053,#9054) ;
#7761=AXIS2_PLACEMENT_3D('',#11692,#9058,#9059) ;
#7762=AXIS2_PLACEMENT_3D('',#11698,#9063,#9064) ;
#7763=AXIS2_PLACEMENT_3D('',#11704,#9068,#9069) ;
#7764=AXIS2_PLACEMENT_3D('',#11710,#9073,#9074) ;
#7765=AXIS2_PLACEMENT_3D('',#11713,#9075,#9076) ;
#7766=AXIS2_PLACEMENT_3D('',#11716,#9079,#9080) ;
#7767=AXIS2_PLACEMENT_3D('',#11720,#9083,#9084) ;
#7768=AXIS2_PLACEMENT_3D('',#11722,#9085,#9086) ;
#7769=AXIS2_PLACEMENT_3D('',#11724,#9088,#9089) ;
#7770=AXIS2_PLACEMENT_3D('',#11726,#9091,#9092) ;
#7771=AXIS2_PLACEMENT_3D('',#11728,#9093,#9094) ;
#7772=AXIS2_PLACEMENT_3D('',#11730,#9095,#9096) ;
#7773=AXIS2_PLACEMENT_3D('',#11732,#9098,#9099) ;
#7774=AXIS2_PLACEMENT_3D('',#11737,#9101,#9102) ;
#7775=AXIS2_PLACEMENT_3D('',#11741,#9104,#9105) ;
#7776=AXIS2_PLACEMENT_3D('',#11744,#9107,#9108) ;
#7777=AXIS2_PLACEMENT_3D('',#11745,#9109,#9110) ;
#7778=AXIS2_PLACEMENT_3D('',#11748,#9111,#9112) ;
#7779=AXIS2_PLACEMENT_3D('',#11752,#9114,#9115) ;
#7780=AXIS2_PLACEMENT_3D('',#11754,#9117,#9118) ;
#7781=AXIS2_PLACEMENT_3D('',#11758,#9120,#9121) ;
#7782=AXIS2_PLACEMENT_3D('',#11760,#9122,#9123) ;
#7783=AXIS2_PLACEMENT_3D('',#11763,#9125,#9126) ;
#7784=AXIS2_PLACEMENT_3D('',#11764,#9127,#9128) ;
#7785=AXIS2_PLACEMENT_3D('',#11767,#9129,#9130) ;
#7786=AXIS2_PLACEMENT_3D('',#11771,#9132,#9133) ;
#7787=AXIS2_PLACEMENT_3D('',#11773,#9135,#9136) ;
#7788=AXIS2_PLACEMENT_3D('',#11777,#9138,#9139) ;
#7789=AXIS2_PLACEMENT_3D('',#11779,#9140,#9141) ;
#7790=AXIS2_PLACEMENT_3D('',#11782,#9143,#9144) ;
#7791=AXIS2_PLACEMENT_3D('',#11783,#9145,#9146) ;
#7792=AXIS2_PLACEMENT_3D('',#11786,#9147,#9148) ;
#7793=AXIS2_PLACEMENT_3D('',#11790,#9150,#9151) ;
#7794=AXIS2_PLACEMENT_3D('',#11792,#9153,#9154) ;
#7795=AXIS2_PLACEMENT_3D('',#11796,#9156,#9157) ;
#7796=AXIS2_PLACEMENT_3D('',#11798,#9158,#9159) ;
#7797=AXIS2_PLACEMENT_3D('',#11801,#9161,#9162) ;
#7798=AXIS2_PLACEMENT_3D('',#11802,#9163,#9164) ;
#7799=AXIS2_PLACEMENT_3D('',#11805,#9165,#9166) ;
#7800=AXIS2_PLACEMENT_3D('',#11809,#9168,#9169) ;
#7801=AXIS2_PLACEMENT_3D('',#11811,#9171,#9172) ;
#7802=AXIS2_PLACEMENT_3D('',#11815,#9174,#9175) ;
#7803=AXIS2_PLACEMENT_3D('',#11817,#9176,#9177) ;
#7804=AXIS2_PLACEMENT_3D('',#11820,#9179,#9180) ;
#7805=AXIS2_PLACEMENT_3D('',#11821,#9181,#9182) ;
#7806=AXIS2_PLACEMENT_3D('',#11824,#9183,#9184) ;
#7807=AXIS2_PLACEMENT_3D('',#11828,#9186,#9187) ;
#7808=AXIS2_PLACEMENT_3D('',#11830,#9189,#9190) ;
#7809=AXIS2_PLACEMENT_3D('',#11834,#9192,#9193) ;
#7810=AXIS2_PLACEMENT_3D('',#11836,#9194,#9195) ;
#7811=AXIS2_PLACEMENT_3D('',#11839,#9197,#9198) ;
#7812=AXIS2_PLACEMENT_3D('',#11840,#9199,#9200) ;
#7813=AXIS2_PLACEMENT_3D('',#11843,#9201,#9202) ;
#7814=AXIS2_PLACEMENT_3D('',#11847,#9204,#9205) ;
#7815=AXIS2_PLACEMENT_3D('',#11849,#9207,#9208) ;
#7816=AXIS2_PLACEMENT_3D('',#11851,#9209,#9210) ;
#7817=AXIS2_PLACEMENT_3D('',#11854,#9212,#9213) ;
#7818=AXIS2_PLACEMENT_3D('',#11855,#9214,#9215) ;
#7819=AXIS2_PLACEMENT_3D('',#11857,#9216,#9217) ;
#7820=AXIS2_PLACEMENT_3D('',#11860,#9219,#9220) ;
#7821=AXIS2_PLACEMENT_3D('',#11861,#9221,#9222) ;
#7822=AXIS2_PLACEMENT_3D('',#11863,#9223,#9224) ;
#7823=AXIS2_PLACEMENT_3D('',#11866,#9226,#9227) ;
#7824=AXIS2_PLACEMENT_3D('',#11867,#9228,#9229) ;
#7825=AXIS2_PLACEMENT_3D('',#11869,#9230,#9231) ;
#7826=AXIS2_PLACEMENT_3D('',#11872,#9233,#9234) ;
#7827=AXIS2_PLACEMENT_3D('',#11873,#9235,#9236) ;
#7828=AXIS2_PLACEMENT_3D('',#11875,#9237,#9238) ;
#7829=AXIS2_PLACEMENT_3D('',#11878,#9240,#9241) ;
#7830=AXIS2_PLACEMENT_3D('',#11879,#9242,#9243) ;
#7831=AXIS2_PLACEMENT_3D('',#11881,#9244,#9245) ;
#7832=AXIS2_PLACEMENT_3D('',#11884,#9247,#9248) ;
#7833=AXIS2_PLACEMENT_3D('',#11885,#9249,#9250) ;
#7834=AXIS2_PLACEMENT_3D('',#11887,#9251,#9252) ;
#7835=AXIS2_PLACEMENT_3D('',#11890,#9254,#9255) ;
#7836=AXIS2_PLACEMENT_3D('',#11891,#9256,#9257) ;
#7837=AXIS2_PLACEMENT_3D('',#11892,#9258,#9259) ;
#7838=AXIS2_PLACEMENT_3D('',#11894,#9260,#9261) ;
#7839=AXIS2_PLACEMENT_3D('',#11897,#9263,#9264) ;
#7840=AXIS2_PLACEMENT_3D('',#11898,#9265,#9266) ;
#7841=AXIS2_PLACEMENT_3D('',#11899,#9267,#9268) ;
#7842=AXIS2_PLACEMENT_3D('',#11900,#9269,#9270) ;
#7843=AXIS2_PLACEMENT_3D('',#11901,#9271,#9272) ;
#7844=AXIS2_PLACEMENT_3D('',#11902,#9273,#9274) ;
#7845=AXIS2_PLACEMENT_3D('',#11903,#9275,#9276) ;
#7846=AXIS2_PLACEMENT_3D('',#11904,#9277,#9278) ;
#7847=AXIS2_PLACEMENT_3D('',#11905,#9279,#9280) ;
#7848=AXIS2_PLACEMENT_3D('',#11906,#9281,#9282) ;
#7849=AXIS2_PLACEMENT_3D('',#11907,#9283,#9284) ;
#7850=AXIS2_PLACEMENT_3D('',#11908,#9285,#9286) ;
#7851=AXIS2_PLACEMENT_3D('',#11909,#9287,#9288) ;
#7852=AXIS2_PLACEMENT_3D('',#11910,#9289,#9290) ;
#7853=AXIS2_PLACEMENT_3D('',#11911,#9291,#9292) ;
#7854=AXIS2_PLACEMENT_3D('',#11912,#9293,#9294) ;
#7855=AXIS2_PLACEMENT_3D('',#11913,#9295,#9296) ;
#7856=AXIS2_PLACEMENT_3D('',#11914,#9297,#9298) ;
#7857=AXIS2_PLACEMENT_3D('',#11915,#9299,#9300) ;
#7858=AXIS2_PLACEMENT_3D('',#11916,#9301,#9302) ;
#7859=AXIS2_PLACEMENT_3D('',#11917,#9303,#9304) ;
#7860=AXIS2_PLACEMENT_3D('',#11918,#9305,#9306) ;
#7861=AXIS2_PLACEMENT_3D('',#11921,#9309,#9310) ;
#7862=AXIS2_PLACEMENT_3D('',#11922,#9311,#9312) ;
#7863=AXIS2_PLACEMENT_3D('',#11924,#9314,#9315) ;
#7864=AXIS2_PLACEMENT_3D('',#11926,#9317,#9318) ;
#7865=AXIS2_PLACEMENT_3D('',#11927,#9319,#9320) ;
#7866=AXIS2_PLACEMENT_3D('',#11929,#9322,#9323) ;
#7867=AXIS2_PLACEMENT_3D('',#11931,#9325,#9326) ;
#7868=AXIS2_PLACEMENT_3D('',#11932,#9327,#9328) ;
#7869=AXIS2_PLACEMENT_3D('',#11934,#9330,#9331) ;
#7870=AXIS2_PLACEMENT_3D('',#11936,#9333,#9334) ;
#7871=AXIS2_PLACEMENT_3D('',#11937,#9335,#9336) ;
#7872=AXIS2_PLACEMENT_3D('',#11938,#9337,#9338) ;
#7873=AXIS2_PLACEMENT_3D('',#11939,#9339,#9340) ;
#7874=AXIS2_PLACEMENT_3D('',#11940,#9341,#9342) ;
#7875=AXIS2_PLACEMENT_3D('',#11941,#9343,#9344) ;
#7876=AXIS2_PLACEMENT_3D('',#11943,#9345,#9346) ;
#7877=AXIS2_PLACEMENT_3D('',#11945,#9348,#9349) ;
#7878=AXIS2_PLACEMENT_3D('',#11947,#9351,#9352) ;
#7879=AXIS2_PLACEMENT_3D('',#11948,#9353,#9354) ;
#7880=AXIS2_PLACEMENT_3D('',#11950,#9356,#9357) ;
#7881=AXIS2_PLACEMENT_3D('',#11952,#9359,#9360) ;
#7882=AXIS2_PLACEMENT_3D('',#11953,#9361,#9362) ;
#7883=AXIS2_PLACEMENT_3D('',#11955,#9364,#9365) ;
#7884=AXIS2_PLACEMENT_3D('',#11957,#9367,#9368) ;
#7885=AXIS2_PLACEMENT_3D('',#11958,#9369,#9370) ;
#7886=AXIS2_PLACEMENT_3D('',#11959,#9371,#9372) ;
#7887=AXIS2_PLACEMENT_3D('',#11961,#9374,#9375) ;
#7888=AXIS2_PLACEMENT_3D('',#11962,#9376,#9377) ;
#7889=AXIS2_PLACEMENT_3D('',#11963,#9378,#9379) ;
#7890=AXIS2_PLACEMENT_3D('',#11964,#9380,#9381) ;
#7891=AXIS2_PLACEMENT_3D('',#11965,#9382,#9383) ;
#7892=AXIS2_PLACEMENT_3D('',#11966,#9384,#9385) ;
#8933=DIRECTION('axis',(0.,0.,1.)) ;
#8934=DIRECTION('refdir',(1.,0.,0.)) ;
#8935=DIRECTION('center_axis',(0.,0.,1.)) ;
#8936=DIRECTION('ref_axis',(1.,0.,0.)) ;
#8937=DIRECTION('',(0.,0.,1.)) ;
#8938=DIRECTION('center_axis',(0.,0.,1.)) ;
#8939=DIRECTION('ref_axis',(-1.,0.,0.)) ;
#8940=DIRECTION('',(0.,0.,1.)) ;
#8941=DIRECTION('center_axis',(0.,0.,1.)) ;
#8942=DIRECTION('ref_axis',(-1.,0.,0.)) ;
#8943=DIRECTION('center_axis',(0.,0.,1.)) ;
#8944=DIRECTION('ref_axis',(1.,0.,0.)) ;
#8945=DIRECTION('center_axis',(0.,0.,1.)) ;
#8946=DIRECTION('ref_axis',(-1.,0.,0.)) ;
#8947=DIRECTION('',(-0.707106781186548,-0.707106781186548,0.)) ;
#8948=DIRECTION('center_axis',(0.,0.,1.)) ;
#8949=DIRECTION('ref_axis',(-1.,0.,0.)) ;
#8950=DIRECTION('',(0.707106781186548,0.707106781186548,0.)) ;
#8951=DIRECTION('center_axis',(0.,0.,1.)) ;
#8952=DIRECTION('ref_axis',(-1.,0.,0.)) ;
#8953=DIRECTION('center_axis',(-0.707106781186548,0.707106781186548,0.)) ;
#8954=DIRECTION('ref_axis',(-0.707106781186548,-0.707106781186548,0.)) ;
#8955=DIRECTION('',(0.,0.,-1.)) ;
#8956=DIRECTION('',(-0.707106781186548,-0.707106781186548,0.)) ;
#8957=DIRECTION('',(0.,0.,1.)) ;
#8958=DIRECTION('center_axis',(0.,0.,1.)) ;
#8959=DIRECTION('ref_axis',(0.479425538604204,-0.877582561890372,0.)) ;
#8960=DIRECTION('center_axis',(0.,0.,1.)) ;
#8961=DIRECTION('ref_axis',(-1.,0.,0.)) ;
#8962=DIRECTION('',(0.,0.,1.)) ;
#8963=DIRECTION('center_axis',(0.,0.,1.)) ;
#8964=DIRECTION('ref_axis',(-1.,0.,0.)) ;
#8965=DIRECTION('',(0.,0.,1.)) ;
#8966=DIRECTION('center_axis',(0.,0.,1.)) ;
#8967=DIRECTION('ref_axis',(-1.,0.,0.)) ;
#8968=DIRECTION('',(0.,0.,1.)) ;
#8969=DIRECTION('center_axis',(0.,0.,1.)) ;
#8970=DIRECTION('ref_axis',(-1.,0.,0.)) ;
#8971=DIRECTION('',(0.,0.,1.)) ;
#8972=DIRECTION('center_axis',(0.,0.,1.)) ;
#8973=DIRECTION('ref_axis',(-1.,0.,0.)) ;
#8974=DIRECTION('',(0.,0.,1.)) ;
#8975=DIRECTION('center_axis',(0.,0.,1.)) ;
#8976=DIRECTION('ref_axis',(-1.,0.,0.)) ;
#8977=DIRECTION('',(0.,0.,1.)) ;
#8978=DIRECTION('center_axis',(0.,0.,1.)) ;
#8979=DIRECTION('ref_axis',(-1.,0.,0.)) ;
#8980=DIRECTION('',(0.,0.,1.)) ;
#8981=DIRECTION('center_axis',(0.,0.,1.)) ;
#8982=DIRECTION('ref_axis',(-1.,0.,0.)) ;
#8983=DIRECTION('',(0.,0.,1.)) ;
#8984=DIRECTION('center_axis',(0.,0.,1.)) ;
#8985=DIRECTION('ref_axis',(-1.,0.,0.)) ;
#8986=DIRECTION('',(0.,0.,1.)) ;
#8987=DIRECTION('center_axis',(0.,0.,1.)) ;
#8988=DIRECTION('ref_axis',(-1.,0.,0.)) ;
#8989=DIRECTION('',(0.,0.,1.)) ;
#8990=DIRECTION('center_axis',(0.,0.,1.)) ;
#8991=DIRECTION('ref_axis',(-1.,0.,0.)) ;
#8992=DIRECTION('',(0.,0.,1.)) ;
#8993=DIRECTION('center_axis',(0.,0.,1.)) ;
#8994=DIRECTION('ref_axis',(-1.,0.,0.)) ;
#8995=DIRECTION('',(0.,0.,1.)) ;
#8996=DIRECTION('center_axis',(0.,0.,1.)) ;
#8997=DIRECTION('ref_axis',(-1.,0.,0.)) ;
#8998=DIRECTION('',(0.,0.,1.)) ;
#8999=DIRECTION('center_axis',(0.,0.,1.)) ;
#9000=DIRECTION('ref_axis',(-1.,0.,0.)) ;
#9001=DIRECTION('',(0.,0.,1.)) ;
#9002=DIRECTION('center_axis',(0.,0.,1.)) ;
#9003=DIRECTION('ref_axis',(-1.,0.,0.)) ;
#9004=DIRECTION('',(0.,0.,1.)) ;
#9005=DIRECTION('center_axis',(0.,0.,1.)) ;
#9006=DIRECTION('ref_axis',(-1.,0.,0.)) ;
#9007=DIRECTION('',(0.,0.,-1.)) ;
#9008=DIRECTION('center_axis',(0.,0.,1.)) ;
#9009=DIRECTION('ref_axis',(-1.,0.,0.)) ;
#9010=DIRECTION('center_axis',(0.707106781186548,-0.707106781186548,0.)) ;
#9011=DIRECTION('ref_axis',(0.707106781186548,0.707106781186548,0.)) ;
#9012=DIRECTION('',(0.,0.,-1.)) ;
#9013=DIRECTION('',(0.707106781186548,0.707106781186548,0.)) ;
#9014=DIRECTION('center_axis',(0.,0.,1.)) ;
#9015=DIRECTION('ref_axis',(1.,0.,0.)) ;
#9016=DIRECTION('center_axis',(0.,0.,1.)) ;
#9017=DIRECTION('ref_axis',(-1.,0.,0.)) ;
#9018=DIRECTION('center_axis',(0.,0.,1.)) ;
#9019=DIRECTION('ref_axis',(-1.,0.,0.)) ;
#9020=DIRECTION('',(1.,0.,0.)) ;
#9021=DIRECTION('center_axis',(0.,0.,1.)) ;
#9022=DIRECTION('ref_axis',(-1.,0.,0.)) ;
#9023=DIRECTION('center_axis',(7.04481399828E-16,-1.,0.)) ;
#9024=DIRECTION('ref_axis',(1.,7.04481399828E-16,0.)) ;
#9025=DIRECTION('',(0.,0.,-1.)) ;
#9026=DIRECTION('',(1.,7.01109518169E-16,0.)) ;
#9027=DIRECTION('center_axis',(-0.707106781186548,-0.707106781186548,0.)) ;
#9028=DIRECTION('ref_axis',(0.707106781186548,-0.707106781186548,0.)) ;
#9029=DIRECTION('',(0.,0.,-1.)) ;
#9030=DIRECTION('',(0.707106781186548,-0.707106781186548,0.)) ;
#9031=DIRECTION('',(0.707106781186548,-0.707106781186548,0.)) ;
#9032=DIRECTION('center_axis',(0.,0.,1.)) ;
#9033=DIRECTION('ref_axis',(1.,0.,0.)) ;
#9034=DIRECTION('',(-1.,0.,0.)) ;
#9035=DIRECTION('center_axis',(0.,0.,1.)) ;
#9036=DIRECTION('ref_axis',(-1.,0.,0.)) ;
#9037=DIRECTION('',(-1.,0.,0.)) ;
#9038=DIRECTION('center_axis',(0.,0.,1.)) ;
#9039=DIRECTION('ref_axis',(-1.,0.,0.)) ;
#9040=DIRECTION('center_axis',(1.,0.,0.)) ;
#9041=DIRECTION('ref_axis',(0.,1.,0.)) ;
#9042=DIRECTION('',(0.,0.,-1.)) ;
#9043=DIRECTION('',(0.,1.,0.)) ;
#9044=DIRECTION('',(0.,1.,0.)) ;
#9045=DIRECTION('center_axis',(0.,0.,-1.)) ;
#9046=DIRECTION('ref_axis',(-2.83106871279E-15,-1.,0.)) ;
#9047=DIRECTION('center_axis',(0.,0.,-1.)) ;
#9048=DIRECTION('ref_axis',(1.,0.,0.)) ;
#9049=DIRECTION('',(0.,0.,-1.)) ;
#9050=DIRECTION('center_axis',(0.,0.,-1.)) ;
#9051=DIRECTION('ref_axis',(1.,0.,0.)) ;
#9052=DIRECTION('',(0.,0.,-1.)) ;
#9053=DIRECTION('center_axis',(-1.,-3.21624529935E-16,0.)) ;
#9054=DIRECTION('ref_axis',(3.21624529935E-16,-1.,0.)) ;
#9055=DIRECTION('',(0.,0.,-1.)) ;
#9056=DIRECTION('',(3.25768058947E-16,-1.,0.)) ;
#9057=DIRECTION('',(3.25768058947E-16,-1.,0.)) ;
#9058=DIRECTION('center_axis',(-0.707106781186548,0.707106781186548,0.)) ;
#9059=DIRECTION('ref_axis',(-0.707106781186548,-0.707106781186548,0.)) ;
#9060=DIRECTION('',(0.,0.,-1.)) ;
#9061=DIRECTION('',(-0.707106781186548,-0.707106781186548,0.)) ;
#9062=DIRECTION('',(-0.707106781186548,-0.707106781186548,0.)) ;
#9063=DIRECTION('center_axis',(-1.60812264968E-16,1.,0.)) ;
#9064=DIRECTION('ref_axis',(-1.,-1.60812264968E-16,0.)) ;
#9065=DIRECTION('',(0.,0.,-1.)) ;
#9066=DIRECTION('',(-1.,-1.55802115149E-16,0.)) ;
#9067=DIRECTION('',(-1.,-1.55802115149E-16,0.)) ;
#9068=DIRECTION('center_axis',(0.707106781186548,0.707106781186548,0.)) ;
#9069=DIRECTION('ref_axis',(-0.707106781186548,0.707106781186548,0.)) ;
#9070=DIRECTION('',(0.,0.,-1.)) ;
#9071=DIRECTION('',(-0.707106781186548,0.707106781186548,0.)) ;
#9072=DIRECTION('',(-0.707106781186548,0.707106781186548,0.)) ;
#9073=DIRECTION('center_axis',(0.,0.,1.)) ;
#9074=DIRECTION('ref_axis',(0.479425538604203,-0.877582561890372,0.)) ;
#9075=DIRECTION('center_axis',(0.,0.,1.)) ;
#9076=DIRECTION('ref_axis',(-1.,0.,0.)) ;
#9077=DIRECTION('',(0.,0.,1.)) ;
#9078=DIRECTION('',(0.,0.,1.)) ;
#9079=DIRECTION('center_axis',(0.,1.,0.)) ;
#9080=DIRECTION('ref_axis',(-1.,0.,0.)) ;
#9081=DIRECTION('',(-1.,0.,0.)) ;
#9082=DIRECTION('',(0.,0.,1.)) ;
#9083=DIRECTION('center_axis',(0.,0.,1.)) ;
#9084=DIRECTION('ref_axis',(0.479425538604203,-0.877582561890372,0.)) ;
#9085=DIRECTION('center_axis',(0.,0.,1.)) ;
#9086=DIRECTION('ref_axis',(-1.,0.,0.)) ;
#9087=DIRECTION('',(0.,0.,1.)) ;
#9088=DIRECTION('center_axis',(0.,1.,0.)) ;
#9089=DIRECTION('ref_axis',(-1.,0.,0.)) ;
#9090=DIRECTION('',(-1.,0.,0.)) ;
#9091=DIRECTION('center_axis',(0.,0.,1.)) ;
#9092=DIRECTION('ref_axis',(1.,0.,0.)) ;
#9093=DIRECTION('center_axis',(0.,0.,1.)) ;
#9094=DIRECTION('ref_axis',(-1.,0.,0.)) ;
#9095=DIRECTION('center_axis',(0.,0.,1.)) ;
#9096=DIRECTION('ref_axis',(-1.,0.,0.)) ;
#9097=DIRECTION('',(0.,0.,1.)) ;
#9098=DIRECTION('center_axis',(0.,0.,-1.)) ;
#9099=DIRECTION('ref_axis',(-0.204112222228953,-0.978947496414776,0.)) ;
#9100=DIRECTION('',(0.,0.,-1.)) ;
#9101=DIRECTION('center_axis',(0.,0.,-1.)) ;
#9102=DIRECTION('ref_axis',(1.,0.,0.)) ;
#9103=DIRECTION('',(0.,0.,-1.)) ;
#9104=DIRECTION('center_axis',(0.,0.,-1.)) ;
#9105=DIRECTION('ref_axis',(1.,0.,0.)) ;
#9106=DIRECTION('',(0.,0.,-1.)) ;
#9107=DIRECTION('center_axis',(0.,0.,-1.)) ;
#9108=DIRECTION('ref_axis',(1.,0.,0.)) ;
#9109=DIRECTION('center_axis',(0.,0.,1.)) ;
#9110=DIRECTION('ref_axis',(-0.382683432365643,0.923879532511058,0.)) ;
#9111=DIRECTION('center_axis',(0.,0.,1.)) ;
#9112=DIRECTION('ref_axis',(-1.,0.,0.)) ;
#9113=DIRECTION('',(0.,0.,1.)) ;
#9114=DIRECTION('center_axis',(0.,0.,1.)) ;
#9115=DIRECTION('ref_axis',(-1.,0.,0.)) ;
#9116=DIRECTION('',(0.,0.,1.)) ;
#9117=DIRECTION('center_axis',(0.,0.,-1.)) ;
#9118=DIRECTION('ref_axis',(0.54789127667893,-0.836549549601894,0.)) ;
#9119=DIRECTION('',(0.,0.,-1.)) ;
#9120=DIRECTION('center_axis',(0.,0.,-1.)) ;
#9121=DIRECTION('ref_axis',(1.,0.,0.)) ;
#9122=DIRECTION('center_axis',(0.,0.,-1.)) ;
#9123=DIRECTION('ref_axis',(1.,0.,0.)) ;
#9124=DIRECTION('',(0.,0.,-1.)) ;
#9125=DIRECTION('center_axis',(0.,0.,-1.)) ;
#9126=DIRECTION('ref_axis',(1.,0.,0.)) ;
#9127=DIRECTION('center_axis',(0.,0.,1.)) ;
#9128=DIRECTION('ref_axis',(0.479425538604203,-0.877582561890372,0.)) ;
#9129=DIRECTION('center_axis',(0.,0.,1.)) ;
#9130=DIRECTION('ref_axis',(-1.,0.,0.)) ;
#9131=DIRECTION('',(0.,0.,1.)) ;
#9132=DIRECTION('center_axis',(0.,0.,1.)) ;
#9133=DIRECTION('ref_axis',(-1.,0.,0.)) ;
#9134=DIRECTION('',(0.,0.,1.)) ;
#9135=DIRECTION('center_axis',(0.,0.,-1.)) ;
#9136=DIRECTION('ref_axis',(0.978947496414776,-0.204112222228953,0.)) ;
#9137=DIRECTION('',(0.,0.,-1.)) ;
#9138=DIRECTION('center_axis',(0.,0.,-1.)) ;
#9139=DIRECTION('ref_axis',(1.,0.,0.)) ;
#9140=DIRECTION('center_axis',(0.,0.,-1.)) ;
#9141=DIRECTION('ref_axis',(1.,0.,0.)) ;
#9142=DIRECTION('',(0.,0.,-1.)) ;
#9143=DIRECTION('center_axis',(0.,0.,-1.)) ;
#9144=DIRECTION('ref_axis',(1.,0.,0.)) ;
#9145=DIRECTION('center_axis',(0.,0.,1.)) ;
#9146=DIRECTION('ref_axis',(0.479425538604203,-0.877582561890372,0.)) ;
#9147=DIRECTION('center_axis',(0.,0.,1.)) ;
#9148=DIRECTION('ref_axis',(-1.,0.,0.)) ;
#9149=DIRECTION('',(0.,0.,1.)) ;
#9150=DIRECTION('center_axis',(0.,0.,1.)) ;
#9151=DIRECTION('ref_axis',(-1.,0.,0.)) ;
#9152=DIRECTION('',(0.,0.,1.)) ;
#9153=DIRECTION('center_axis',(0.,0.,-1.)) ;
#9154=DIRECTION('ref_axis',(0.836549549601894,0.54789127667893,0.)) ;
#9155=DIRECTION('',(0.,0.,-1.)) ;
#9156=DIRECTION('center_axis',(0.,0.,-1.)) ;
#9157=DIRECTION('ref_axis',(1.,0.,0.)) ;
#9158=DIRECTION('center_axis',(0.,0.,-1.)) ;
#9159=DIRECTION('ref_axis',(1.,0.,0.)) ;
#9160=DIRECTION('',(0.,0.,-1.)) ;
#9161=DIRECTION('center_axis',(0.,0.,-1.)) ;
#9162=DIRECTION('ref_axis',(1.,0.,0.)) ;
#9163=DIRECTION('center_axis',(0.,0.,1.)) ;
#9164=DIRECTION('ref_axis',(0.479425538604203,-0.877582561890372,0.)) ;
#9165=DIRECTION('center_axis',(0.,0.,1.)) ;
#9166=DIRECTION('ref_axis',(-1.,0.,0.)) ;
#9167=DIRECTION('',(0.,0.,1.)) ;
#9168=DIRECTION('center_axis',(0.,0.,1.)) ;
#9169=DIRECTION('ref_axis',(-1.,0.,0.)) ;
#9170=DIRECTION('',(0.,0.,1.)) ;
#9171=DIRECTION('center_axis',(0.,0.,-1.)) ;
#9172=DIRECTION('ref_axis',(0.204112222228953,0.978947496414776,0.)) ;
#9173=DIRECTION('',(0.,0.,-1.)) ;
#9174=DIRECTION('center_axis',(0.,0.,-1.)) ;
#9175=DIRECTION('ref_axis',(1.,0.,0.)) ;
#9176=DIRECTION('center_axis',(0.,0.,-1.)) ;
#9177=DIRECTION('ref_axis',(1.,0.,0.)) ;
#9178=DIRECTION('',(0.,0.,-1.)) ;
#9179=DIRECTION('center_axis',(0.,0.,-1.)) ;
#9180=DIRECTION('ref_axis',(1.,0.,0.)) ;
#9181=DIRECTION('center_axis',(0.,0.,1.)) ;
#9182=DIRECTION('ref_axis',(0.479425538604203,-0.877582561890372,0.)) ;
#9183=DIRECTION('center_axis',(0.,0.,1.)) ;
#9184=DIRECTION('ref_axis',(-1.,0.,0.)) ;
#9185=DIRECTION('',(0.,0.,1.)) ;
#9186=DIRECTION('center_axis',(0.,0.,1.)) ;
#9187=DIRECTION('ref_axis',(-1.,0.,0.)) ;
#9188=DIRECTION('',(0.,0.,1.)) ;
#9189=DIRECTION('center_axis',(0.,0.,-1.)) ;
#9190=DIRECTION('ref_axis',(-0.54789127667893,0.836549549601894,0.)) ;
#9191=DIRECTION('',(0.,0.,-1.)) ;
#9192=DIRECTION('center_axis',(0.,0.,-1.)) ;
#9193=DIRECTION('ref_axis',(1.,0.,0.)) ;
#9194=DIRECTION('center_axis',(0.,0.,-1.)) ;
#9195=DIRECTION('ref_axis',(1.,0.,0.)) ;
#9196=DIRECTION('',(0.,0.,-1.)) ;
#9197=DIRECTION('center_axis',(0.,0.,-1.)) ;
#9198=DIRECTION('ref_axis',(1.,0.,0.)) ;
#9199=DIRECTION('center_axis',(0.,0.,1.)) ;
#9200=DIRECTION('ref_axis',(0.479425538604203,-0.877582561890372,0.)) ;
#9201=DIRECTION('center_axis',(0.,0.,1.)) ;
#9202=DIRECTION('ref_axis',(-1.,0.,0.)) ;
#9203=DIRECTION('',(0.,0.,1.)) ;
#9204=DIRECTION('center_axis',(0.,0.,1.)) ;
#9205=DIRECTION('ref_axis',(-1.,0.,0.)) ;
#9206=DIRECTION('',(0.,0.,1.)) ;
#9207=DIRECTION('center_axis',(0.,0.,1.)) ;
#9208=DIRECTION('ref_axis',(-1.,1.22464679914735E-16,0.)) ;
#9209=DIRECTION('center_axis',(0.,0.,1.)) ;
#9210=DIRECTION('ref_axis',(-1.,0.,0.)) ;
#9211=DIRECTION('',(0.,0.,1.)) ;
#9212=DIRECTION('center_axis',(0.,0.,1.)) ;
#9213=DIRECTION('ref_axis',(-1.,0.,0.)) ;
#9214=DIRECTION('center_axis',(0.,0.,1.)) ;
#9215=DIRECTION('ref_axis',(1.,0.,0.)) ;
#9216=DIRECTION('center_axis',(0.,0.,1.)) ;
#9217=DIRECTION('ref_axis',(-1.,0.,0.)) ;
#9218=DIRECTION('',(0.,0.,1.)) ;
#9219=DIRECTION('center_axis',(0.,0.,1.)) ;
#9220=DIRECTION('ref_axis',(-1.,0.,0.)) ;
#9221=DIRECTION('center_axis',(0.,0.,1.)) ;
#9222=DIRECTION('ref_axis',(1.,0.,0.)) ;
#9223=DIRECTION('center_axis',(0.,0.,1.)) ;
#9224=DIRECTION('ref_axis',(-1.,0.,0.)) ;
#9225=DIRECTION('',(0.,0.,1.)) ;
#9226=DIRECTION('center_axis',(0.,0.,1.)) ;
#9227=DIRECTION('ref_axis',(-1.,0.,0.)) ;
#9228=DIRECTION('center_axis',(0.,0.,1.)) ;
#9229=DIRECTION('ref_axis',(1.,0.,0.)) ;
#9230=DIRECTION('center_axis',(0.,0.,1.)) ;
#9231=DIRECTION('ref_axis',(-1.,0.,0.)) ;
#9232=DIRECTION('',(0.,0.,1.)) ;
#9233=DIRECTION('center_axis',(0.,0.,1.)) ;
#9234=DIRECTION('ref_axis',(-1.,0.,0.)) ;
#9235=DIRECTION('center_axis',(0.,0.,1.)) ;
#9236=DIRECTION('ref_axis',(1.,0.,0.)) ;
#9237=DIRECTION('center_axis',(0.,0.,1.)) ;
#9238=DIRECTION('ref_axis',(-1.,0.,0.)) ;
#9239=DIRECTION('',(0.,0.,1.)) ;
#9240=DIRECTION('center_axis',(0.,0.,1.)) ;
#9241=DIRECTION('ref_axis',(-1.,0.,0.)) ;
#9242=DIRECTION('center_axis',(0.,0.,1.)) ;
#9243=DIRECTION('ref_axis',(1.,0.,0.)) ;
#9244=DIRECTION('center_axis',(0.,0.,1.)) ;
#9245=DIRECTION('ref_axis',(-1.,0.,0.)) ;
#9246=DIRECTION('',(0.,0.,1.)) ;
#9247=DIRECTION('center_axis',(0.,0.,1.)) ;
#9248=DIRECTION('ref_axis',(-1.,0.,0.)) ;
#9249=DIRECTION('center_axis',(0.,0.,1.)) ;
#9250=DIRECTION('ref_axis',(0.479425538604203,-0.877582561890372,0.)) ;
#9251=DIRECTION('center_axis',(0.,0.,1.)) ;
#9252=DIRECTION('ref_axis',(-1.,0.,0.)) ;
#9253=DIRECTION('',(0.,0.,1.)) ;
#9254=DIRECTION('center_axis',(0.,0.,1.)) ;
#9255=DIRECTION('ref_axis',(-1.,0.,0.)) ;
#9256=DIRECTION('center_axis',(0.,0.,-1.)) ;
#9257=DIRECTION('ref_axis',(-0.978947496414776,0.204112222228953,0.)) ;
#9258=DIRECTION('center_axis',(0.,0.,-1.)) ;
#9259=DIRECTION('ref_axis',(1.,0.,0.)) ;
#9260=DIRECTION('center_axis',(0.,0.,-1.)) ;
#9261=DIRECTION('ref_axis',(1.,0.,0.)) ;
#9262=DIRECTION('',(0.,0.,-1.)) ;
#9263=DIRECTION('center_axis',(0.,0.,-1.)) ;
#9264=DIRECTION('ref_axis',(1.,0.,0.)) ;
#9265=DIRECTION('center_axis',(0.,0.,-1.)) ;
#9266=DIRECTION('ref_axis',(0.707106781186548,0.707106781186548,0.)) ;
#9267=DIRECTION('center_axis',(0.,0.,-1.)) ;
#9268=DIRECTION('ref_axis',(1.,0.,0.)) ;
#9269=DIRECTION('center_axis',(0.,0.,-1.)) ;
#9270=DIRECTION('ref_axis',(1.,0.,0.)) ;
#9271=DIRECTION('center_axis',(0.,0.,-1.)) ;
#9272=DIRECTION('ref_axis',(1.,0.,0.)) ;
#9273=DIRECTION('center_axis',(0.,0.,-1.)) ;
#9274=DIRECTION('ref_axis',(1.88737914186E-15,1.,0.)) ;
#9275=DIRECTION('center_axis',(0.,0.,-1.)) ;
#9276=DIRECTION('ref_axis',(1.,0.,0.)) ;
#9277=DIRECTION('center_axis',(0.,0.,-1.)) ;
#9278=DIRECTION('ref_axis',(1.,0.,0.)) ;
#9279=DIRECTION('center_axis',(0.,0.,-1.)) ;
#9280=DIRECTION('ref_axis',(1.,0.,0.)) ;
#9281=DIRECTION('center_axis',(0.,0.,-1.)) ;
#9282=DIRECTION('ref_axis',(-0.707106781186548,0.707106781186548,0.)) ;
#9283=DIRECTION('center_axis',(0.,0.,-1.)) ;
#9284=DIRECTION('ref_axis',(1.,0.,0.)) ;
#9285=DIRECTION('center_axis',(0.,0.,-1.)) ;
#9286=DIRECTION('ref_axis',(1.,0.,0.)) ;
#9287=DIRECTION('center_axis',(0.,0.,-1.)) ;
#9288=DIRECTION('ref_axis',(1.,0.,0.)) ;
#9289=DIRECTION('center_axis',(0.,0.,-1.)) ;
#9290=DIRECTION('ref_axis',(-1.,-1.52655665886E-15,0.)) ;
#9291=DIRECTION('center_axis',(0.,0.,-1.)) ;
#9292=DIRECTION('ref_axis',(1.,0.,0.)) ;
#9293=DIRECTION('center_axis',(0.,0.,-1.)) ;
#9294=DIRECTION('ref_axis',(1.,0.,0.)) ;
#9295=DIRECTION('center_axis',(0.,0.,-1.)) ;
#9296=DIRECTION('ref_axis',(1.,0.,0.)) ;
#9297=DIRECTION('center_axis',(0.,0.,-1.)) ;
#9298=DIRECTION('ref_axis',(1.,1.94289029309E-16,0.)) ;
#9299=DIRECTION('center_axis',(0.,0.,-1.)) ;
#9300=DIRECTION('ref_axis',(1.,0.,0.)) ;
#9301=DIRECTION('center_axis',(0.,0.,-1.)) ;
#9302=DIRECTION('ref_axis',(1.,0.,0.)) ;
#9303=DIRECTION('center_axis',(0.,0.,-1.)) ;
#9304=DIRECTION('ref_axis',(1.,0.,0.)) ;
#9305=DIRECTION('center_axis',(-0.707106781186548,-0.707106781186548,0.)) ;
#9306=DIRECTION('ref_axis',(0.707106781186548,-0.707106781186548,0.)) ;
#9307=DIRECTION('',(0.707106781186548,-0.707106781186548,0.)) ;
#9308=DIRECTION('',(0.707106781186548,-0.707106781186548,0.)) ;
#9309=DIRECTION('center_axis',(0.,0.,1.)) ;
#9310=DIRECTION('ref_axis',(1.,0.,0.)) ;
#9311=DIRECTION('center_axis',(0.,0.,1.)) ;
#9312=DIRECTION('ref_axis',(1.,0.,0.)) ;
#9313=DIRECTION('',(1.,0.,0.)) ;
#9314=DIRECTION('center_axis',(1.60812264968E-16,-1.,0.)) ;
#9315=DIRECTION('ref_axis',(1.,1.60812264968E-16,0.)) ;
#9316=DIRECTION('',(1.,1.62884029474E-16,0.)) ;
#9317=DIRECTION('center_axis',(0.,0.,1.)) ;
#9318=DIRECTION('ref_axis',(1.,0.,0.)) ;
#9319=DIRECTION('center_axis',(0.,0.,1.)) ;
#9320=DIRECTION('ref_axis',(1.,0.,0.)) ;
#9321=DIRECTION('',(0.707106781186548,0.707106781186548,0.)) ;
#9322=DIRECTION('center_axis',(0.707106781186548,-0.707106781186548,0.)) ;
#9323=DIRECTION('ref_axis',(0.707106781186548,0.707106781186548,0.)) ;
#9324=DIRECTION('',(0.707106781186548,0.707106781186548,0.)) ;
#9325=DIRECTION('center_axis',(0.,0.,1.)) ;
#9326=DIRECTION('ref_axis',(1.,0.,0.)) ;
#9327=DIRECTION('center_axis',(0.,0.,1.)) ;
#9328=DIRECTION('ref_axis',(1.,0.,0.)) ;
#9329=DIRECTION('',(-3.18686144622E-16,1.,0.)) ;
#9330=DIRECTION('center_axis',(1.,3.21624529935E-16,0.)) ;
#9331=DIRECTION('ref_axis',(-3.21624529935E-16,1.,0.)) ;
#9332=DIRECTION('',(-3.18686144622E-16,1.,0.)) ;
#9333=DIRECTION('center_axis',(0.,0.,1.)) ;
#9334=DIRECTION('ref_axis',(1.,0.,0.)) ;
#9335=DIRECTION('center_axis',(0.,0.,-1.)) ;
#9336=DIRECTION('ref_axis',(-0.707106781186548,-0.707106781186548,0.)) ;
#9337=DIRECTION('center_axis',(0.,0.,-1.)) ;
#9338=DIRECTION('ref_axis',(1.,0.,0.)) ;
#9339=DIRECTION('center_axis',(0.,0.,-1.)) ;
#9340=DIRECTION('ref_axis',(1.,0.,0.)) ;
#9341=DIRECTION('center_axis',(0.,0.,-1.)) ;
#9342=DIRECTION('ref_axis',(1.,0.,0.)) ;
#9343=DIRECTION('center_axis',(0.,0.,1.)) ;
#9344=DIRECTION('ref_axis',(0.479425538604203,-0.877582561890372,0.)) ;
#9345=DIRECTION('center_axis',(0.,0.,1.)) ;
#9346=DIRECTION('ref_axis',(-1.,0.,0.)) ;
#9347=DIRECTION('',(0.,0.,1.)) ;
#9348=DIRECTION('center_axis',(0.,0.,1.)) ;
#9349=DIRECTION('ref_axis',(1.,0.,0.)) ;
#9350=DIRECTION('',(0.,-1.,0.)) ;
#9351=DIRECTION('center_axis',(0.,0.,1.)) ;
#9352=DIRECTION('ref_axis',(1.,0.,0.)) ;
#9353=DIRECTION('center_axis',(0.,0.,1.)) ;
#9354=DIRECTION('ref_axis',(1.,0.,0.)) ;
#9355=DIRECTION('',(-0.707106781186548,0.707106781186548,0.)) ;
#9356=DIRECTION('center_axis',(0.707106781186548,0.707106781186548,0.)) ;
#9357=DIRECTION('ref_axis',(-0.707106781186548,0.707106781186548,0.)) ;
#9358=DIRECTION('',(-0.707106781186548,0.707106781186548,0.)) ;
#9359=DIRECTION('center_axis',(0.,0.,1.)) ;
#9360=DIRECTION('ref_axis',(1.,0.,0.)) ;
#9361=DIRECTION('center_axis',(0.,0.,1.)) ;
#9362=DIRECTION('ref_axis',(1.,0.,0.)) ;
#9363=DIRECTION('',(-1.,-9.06485033593E-16,0.)) ;
#9364=DIRECTION('center_axis',(-7.04481399828E-16,1.,0.)) ;
#9365=DIRECTION('ref_axis',(-1.,-7.04481399828E-16,0.)) ;
#9366=DIRECTION('',(-1.,-7.01109518169E-16,0.)) ;
#9367=DIRECTION('center_axis',(0.,0.,1.)) ;
#9368=DIRECTION('ref_axis',(1.,0.,0.)) ;
#9369=DIRECTION('center_axis',(0.,0.,1.)) ;
#9370=DIRECTION('ref_axis',(1.,0.,0.)) ;
#9371=DIRECTION('center_axis',(0.,0.,1.)) ;
#9372=DIRECTION('ref_axis',(-1.,0.,0.)) ;
#9373=DIRECTION('',(0.,-1.,0.)) ;
#9374=DIRECTION('center_axis',(-1.,0.,0.)) ;
#9375=DIRECTION('ref_axis',(0.,-1.,0.)) ;
#9376=DIRECTION('center_axis',(0.,0.,-1.)) ;
#9377=DIRECTION('ref_axis',(-0.836549549601894,-0.54789127667893,0.)) ;
#9378=DIRECTION('center_axis',(0.,0.,-1.)) ;
#9379=DIRECTION('ref_axis',(1.,0.,0.)) ;
#9380=DIRECTION('center_axis',(0.,0.,-1.)) ;
#9381=DIRECTION('ref_axis',(0.707106781186548,-0.707106781186548,0.)) ;
#9382=DIRECTION('center_axis',(0.,0.,-1.)) ;
#9383=DIRECTION('ref_axis',(1.,0.,0.)) ;
#9384=DIRECTION('center_axis',(0.,0.,1.)) ;
#9385=DIRECTION('ref_axis',(1.,0.,0.)) ;
#11550=CARTESIAN_POINT('',(0.,0.,0.)) ;
#11551=CARTESIAN_POINT('Origin',(0.,0.,133.410000002)) ;
#11552=CARTESIAN_POINT('',(5.29728275935,3.93685094555,132.6)) ;
#11553=CARTESIAN_POINT('',(5.29728275935,3.93685094555,132.9)) ;
#11554=CARTESIAN_POINT('',(5.29728275935,3.93685094555,133.410000002)) ;
#11555=CARTESIAN_POINT('',(3.93685094555,5.29728275935,132.9)) ;
#11556=CARTESIAN_POINT('Origin',(0.,0.,132.9)) ;
#11557=CARTESIAN_POINT('',(3.93685094555,5.29728275935,132.6)) ;
#11558=CARTESIAN_POINT('',(3.93685094555,5.29728275935,133.410000002)) ;
#11559=CARTESIAN_POINT('Origin',(0.,0.,132.6)) ;
#11560=CARTESIAN_POINT('Origin',(0.,0.,132.9)) ;
#11561=CARTESIAN_POINT('',(5.41863850166,4.13400319968,132.9)) ;
#11562=CARTESIAN_POINT('Origin',(5.77219189225,3.78044980909,132.9)) ;
#11563=CARTESIAN_POINT('',(16.5038648024,15.2192295004,132.9)) ;
#11564=CARTESIAN_POINT('',(10.961251652,9.67661635003,132.9)) ;
#11565=CARTESIAN_POINT('',(15.2192295004,16.5038648024,132.9)) ;
#11566=CARTESIAN_POINT('Origin',(1.7763568394E-15,-4.4408920985E-16,132.9)) ;
#11567=CARTESIAN_POINT('',(4.13400319968,5.41863850166,132.9)) ;
#11568=CARTESIAN_POINT('',(9.67661635003,10.961251652,132.9)) ;
#11569=CARTESIAN_POINT('Origin',(3.78044980909,5.77219189225,132.9)) ;
#11570=CARTESIAN_POINT('Origin',(16.5038648024,15.2192295004,124.2)) ;
#11571=CARTESIAN_POINT('',(5.41863850166,4.13400319968,124.2)) ;
#11572=CARTESIAN_POINT('',(5.41863850166,4.13400319968,128.55)) ;
#11573=CARTESIAN_POINT('',(16.5038648024,15.2192295004,124.2)) ;
#11574=CARTESIAN_POINT('',(10.961251652,9.67661635003,124.2)) ;
#11575=CARTESIAN_POINT('',(16.5038648024,15.2192295004,128.55)) ;
#11576=CARTESIAN_POINT('Origin',(0.,0.,127.6)) ;
#11577=CARTESIAN_POINT('',(-0.908374333382,22.4316151017,124.2)) ;
#11578=CARTESIAN_POINT('',(-10.7631033416644,19.7017285144389,124.2)) ;
#11579=CARTESIAN_POINT('Origin',(0.,0.,124.2)) ;
#11580=CARTESIAN_POINT('',(-0.908374333382,22.4316151017,132.9)) ;
#11581=CARTESIAN_POINT('',(-0.908374333382,22.4316151017,123.4)) ;
#11582=CARTESIAN_POINT('',(0.908374333382,22.4316151017,132.9)) ;
#11583=CARTESIAN_POINT('Origin',(0.,0.,132.9)) ;
#11584=CARTESIAN_POINT('',(0.908374333382,22.4316151017,124.2)) ;
#11585=CARTESIAN_POINT('',(0.908374333382,22.4316151017,123.4)) ;
#11586=CARTESIAN_POINT('',(15.2192295004,16.5038648024,124.2)) ;
#11587=CARTESIAN_POINT('Origin',(0.,0.,124.2)) ;
#11588=CARTESIAN_POINT('',(15.2192295004,16.5038648024,123.4)) ;
#11589=CARTESIAN_POINT('',(22.4316151017,0.908374333382,124.2)) ;
#11590=CARTESIAN_POINT('Origin',(0.,0.,124.2)) ;
#11591=CARTESIAN_POINT('',(22.4316151017,0.908374333382,132.9)) ;
#11592=CARTESIAN_POINT('',(22.4316151017,0.908374333382,123.4)) ;
#11593=CARTESIAN_POINT('',(22.4316151017,-0.908374333382,132.9)) ;
#11594=CARTESIAN_POINT('Origin',(0.,0.,132.9)) ;
#11595=CARTESIAN_POINT('',(22.4316151017,-0.908374333382,124.2)) ;
#11596=CARTESIAN_POINT('',(22.4316151017,-0.908374333382,123.4)) ;
#11597=CARTESIAN_POINT('',(16.5038648024,-15.2192295004,124.2)) ;
#11598=CARTESIAN_POINT('Origin',(0.,0.,124.2)) ;
#11599=CARTESIAN_POINT('',(16.5038648024,-15.2192295004,132.9)) ;
#11600=CARTESIAN_POINT('',(16.5038648024,-15.2192295004,123.4)) ;
#11601=CARTESIAN_POINT('',(15.2192295004,-16.5038648024,132.9)) ;
#11602=CARTESIAN_POINT('Origin',(0.,0.,132.9)) ;
#11603=CARTESIAN_POINT('',(15.2192295004,-16.5038648024,124.2)) ;
#11604=CARTESIAN_POINT('',(15.2192295004,-16.5038648024,123.4)) ;
#11605=CARTESIAN_POINT('',(0.908374333382,-22.4316151017,124.2)) ;
#11606=CARTESIAN_POINT('Origin',(0.,0.,124.2)) ;
#11607=CARTESIAN_POINT('',(0.908374333382,-22.4316151017,132.9)) ;
#11608=CARTESIAN_POINT('',(0.908374333382,-22.4316151017,123.4)) ;
#11609=CARTESIAN_POINT('',(-0.908374333382,-22.4316151017,132.9)) ;
#11610=CARTESIAN_POINT('Origin',(0.,0.,132.9)) ;
#11611=CARTESIAN_POINT('',(-0.908374333382,-22.4316151017,124.2)) ;
#11612=CARTESIAN_POINT('',(-0.908374333382,-22.4316151017,123.4)) ;
#11613=CARTESIAN_POINT('',(-15.2192295004,-16.5038648024,124.2)) ;
#11614=CARTESIAN_POINT('Origin',(0.,0.,124.2)) ;
#11615=CARTESIAN_POINT('',(-15.2192295004,-16.5038648024,132.9)) ;
#11616=CARTESIAN_POINT('',(-15.2192295004,-16.5038648024,123.4)) ;
#11617=CARTESIAN_POINT('',(-16.5038648024,-15.2192295004,132.9)) ;
#11618=CARTESIAN_POINT('Origin',(0.,0.,132.9)) ;
#11619=CARTESIAN_POINT('',(-16.5038648024,-15.2192295004,124.2)) ;
#11620=CARTESIAN_POINT('',(-16.5038648024,-15.2192295004,123.4)) ;
#11621=CARTESIAN_POINT('',(-22.4316151017,-0.908374333382,124.2)) ;
#11622=CARTESIAN_POINT('Origin',(0.,0.,124.2)) ;
#11623=CARTESIAN_POINT('',(-22.4316151017,-0.908374333382,132.9)) ;
#11624=CARTESIAN_POINT('',(-22.4316151017,-0.908374333382,123.4)) ;
#11625=CARTESIAN_POINT('',(-22.4316151017,0.908374333382,132.9)) ;
#11626=CARTESIAN_POINT('Origin',(0.,0.,132.9)) ;
#11627=CARTESIAN_POINT('',(-22.4316151017,0.908374333382,124.2)) ;
#11628=CARTESIAN_POINT('',(-22.4316151017,0.908374333382,123.4)) ;
#11629=CARTESIAN_POINT('',(-16.5038648024,15.2192295004,124.2)) ;
#11630=CARTESIAN_POINT('Origin',(0.,0.,124.2)) ;
#11631=CARTESIAN_POINT('',(-16.5038648024,15.2192295004,132.9)) ;
#11632=CARTESIAN_POINT('',(-16.5038648024,15.2192295004,123.4)) ;
#11633=CARTESIAN_POINT('',(-15.2192295004,16.5038648024,132.9)) ;
#11634=CARTESIAN_POINT('Origin',(0.,0.,132.9)) ;
#11635=CARTESIAN_POINT('',(-15.2192295004,16.5038648024,124.2)) ;
#11636=CARTESIAN_POINT('',(-15.2192295004,16.5038648024,123.4)) ;
#11637=CARTESIAN_POINT('Origin',(0.,0.,124.2)) ;
#11638=CARTESIAN_POINT('',(-10.7631033417,19.7017285144,122.6)) ;
#11639=CARTESIAN_POINT('',(-10.7631033416644,19.7017285144389,127.6)) ;
#11640=CARTESIAN_POINT('Origin',(0.,0.,122.6)) ;
#11641=CARTESIAN_POINT('Origin',(3.83735064423,5.12198594621,124.2)) ;
#11642=CARTESIAN_POINT('',(4.13400319968,5.41863850166,124.2)) ;
#11643=CARTESIAN_POINT('',(4.13400319968,5.41863850166,128.55)) ;
#11644=CARTESIAN_POINT('',(9.67661635003,10.961251652,124.2)) ;
#11645=CARTESIAN_POINT('Origin',(0.,-22.45,124.2)) ;
#11646=CARTESIAN_POINT('',(6.26526397705,1.30631822227,124.2)) ;
#11647=CARTESIAN_POINT('',(5.35391711745,3.50650417075,124.2)) ;
#11648=CARTESIAN_POINT('Origin',(0.,0.,124.2)) ;
#11649=CARTESIAN_POINT('',(6.75473772526,0.908374333382,124.2)) ;
#11650=CARTESIAN_POINT('Origin',(6.75473772526,1.40837433338,124.2)) ;
#11651=CARTESIAN_POINT('',(14.5931764135,0.908374333382,124.2)) ;
#11652=CARTESIAN_POINT('Origin',(5.77219189225,3.78044980909,124.2)) ;
#11653=CARTESIAN_POINT('Origin',(6.33520765804,0.908374333382,124.2)) ;
#11654=CARTESIAN_POINT('',(6.75473772526,0.908374333382,132.9)) ;
#11655=CARTESIAN_POINT('',(6.75473772526,0.908374333382,128.55)) ;
#11656=CARTESIAN_POINT('',(14.5931764135,0.908374333382,132.9)) ;
#11657=CARTESIAN_POINT('Origin',(5.12198594621,-3.83735064423,124.2)) ;
#11658=CARTESIAN_POINT('',(5.41863850166,-4.13400319968,132.9)) ;
#11659=CARTESIAN_POINT('',(5.41863850166,-4.13400319968,124.2)) ;
#11660=CARTESIAN_POINT('',(5.41863850166,-4.13400319968,128.55)) ;
#11661=CARTESIAN_POINT('',(10.961251652,-9.67661635003,132.9)) ;
#11662=CARTESIAN_POINT('',(10.961251652,-9.67661635003,124.2)) ;
#11663=CARTESIAN_POINT('Origin',(0.,-4.45,122.6)) ;
#11664=CARTESIAN_POINT('',(-2.14301189917,-3.9,122.6)) ;
#11665=CARTESIAN_POINT('',(2.14301189917,-3.9,122.6)) ;
#11666=CARTESIAN_POINT('',(1.7763568394E-15,-3.9,122.6)) ;
#11667=CARTESIAN_POINT('',(2.14301189917,3.9,122.6)) ;
#11668=CARTESIAN_POINT('Origin',(0.,0.,122.6)) ;
#11669=CARTESIAN_POINT('',(-2.14301189917,3.9,122.6)) ;
#11670=CARTESIAN_POINT('',(0.,3.9,122.6)) ;
#11671=CARTESIAN_POINT('Origin',(0.,0.,122.6)) ;
#11672=CARTESIAN_POINT('Origin',(-0.908374333382,6.33520765804,124.2)) ;
#11673=CARTESIAN_POINT('',(-0.908374333382,6.75473772526,132.9)) ;
#11674=CARTESIAN_POINT('',(-0.908374333382,6.75473772526,124.2)) ;
#11675=CARTESIAN_POINT('',(-0.908374333382,6.75473772526,128.55)) ;
#11676=CARTESIAN_POINT('',(-0.908374333382,14.5931764135,132.9)) ;
#11677=CARTESIAN_POINT('',(-0.908374333382,14.5931764135,124.2)) ;
#11678=CARTESIAN_POINT('Origin',(6.75473772526,1.40837433338,128.55)) ;
#11679=CARTESIAN_POINT('',(6.26526397705,1.30631822227,132.6)) ;
#11680=CARTESIAN_POINT('',(6.52951856112,0.961970560881,132.6)) ;
#11681=CARTESIAN_POINT('Origin',(6.75473772526,1.40837433338,132.6)) ;
#11682=CARTESIAN_POINT('',(6.52951856112,0.961970560881,132.9)) ;
#11683=CARTESIAN_POINT('',(6.52951856112,0.961970560881,128.55)) ;
#11684=CARTESIAN_POINT('Origin',(6.75473772526,1.40837433338,132.9)) ;
#11685=CARTESIAN_POINT('',(6.26526397705,1.30631822227,128.55)) ;
#11686=CARTESIAN_POINT('Origin',(0.908374333382,-6.33520765804,124.2)) ;
#11687=CARTESIAN_POINT('',(0.908374333382,-6.75473772526,132.9)) ;
#11688=CARTESIAN_POINT('',(0.908374333382,-6.75473772526,124.2)) ;
#11689=CARTESIAN_POINT('',(0.908374333382,-6.75473772526,128.55)) ;
#11690=CARTESIAN_POINT('',(0.908374333382,-14.5931764135,132.9)) ;
#11691=CARTESIAN_POINT('',(0.908374333382,-14.5931764135,124.2)) ;
#11692=CARTESIAN_POINT('Origin',(-3.83735064423,-5.12198594621,124.2)) ;
#11693=CARTESIAN_POINT('',(-4.13400319968,-5.41863850166,132.9)) ;
#11694=CARTESIAN_POINT('',(-4.13400319968,-5.41863850166,124.2)) ;
#11695=CARTESIAN_POINT('',(-4.13400319968,-5.41863850166,128.55)) ;
#11696=CARTESIAN_POINT('',(-9.67661635003,-10.961251652,132.9)) ;
#11697=CARTESIAN_POINT('',(-9.67661635003,-10.961251652,124.2)) ;
#11698=CARTESIAN_POINT('Origin',(-6.33520765804,-0.908374333382,124.2)) ;
#11699=CARTESIAN_POINT('',(-6.75473772526,-0.908374333382,132.9)) ;
#11700=CARTESIAN_POINT('',(-6.75473772526,-0.908374333382,124.2)) ;
#11701=CARTESIAN_POINT('',(-6.75473772526,-0.908374333382,128.55)) ;
#11702=CARTESIAN_POINT('',(-14.5931764135,-0.908374333382,132.9)) ;
#11703=CARTESIAN_POINT('',(-14.5931764135,-0.908374333382,124.2)) ;
#11704=CARTESIAN_POINT('Origin',(-5.12198594621,3.83735064423,124.2)) ;
#11705=CARTESIAN_POINT('',(-5.41863850166,4.13400319968,132.9)) ;
#11706=CARTESIAN_POINT('',(-5.41863850166,4.13400319968,124.2)) ;
#11707=CARTESIAN_POINT('',(-5.41863850166,4.13400319968,128.55)) ;
#11708=CARTESIAN_POINT('',(-10.961251652,9.67661635003,132.9)) ;
#11709=CARTESIAN_POINT('',(-10.961251652,9.67661635003,124.2)) ;
#11710=CARTESIAN_POINT('Origin',(0.,0.,127.6)) ;
#11711=CARTESIAN_POINT('',(-2.14301189917,3.9,132.6)) ;
#11712=CARTESIAN_POINT('',(-2.14301189917,-3.9,132.6)) ;
#11713=CARTESIAN_POINT('Origin',(0.,0.,132.6)) ;
#11714=CARTESIAN_POINT('',(-2.14301189917,-3.9,127.6)) ;
#11715=CARTESIAN_POINT('',(-2.14301189917,3.9,127.6)) ;
#11716=CARTESIAN_POINT('Origin',(2.14301189917,3.9,122.6)) ;
#11717=CARTESIAN_POINT('',(2.14301189917,3.9,132.6)) ;
#11718=CARTESIAN_POINT('',(0.,3.9,132.6)) ;
#11719=CARTESIAN_POINT('',(2.14301189917,3.9,127.6)) ;
#11720=CARTESIAN_POINT('Origin',(0.,0.,127.6)) ;
#11721=CARTESIAN_POINT('',(2.14301189917,-3.9,132.6)) ;
#11722=CARTESIAN_POINT('Origin',(0.,0.,132.6)) ;
#11723=CARTESIAN_POINT('',(2.14301189917,-3.9,127.6)) ;
#11724=CARTESIAN_POINT('Origin',(2.14301189917,-3.9,122.6)) ;
#11725=CARTESIAN_POINT('',(1.7763568394E-15,-3.9,132.6)) ;
#11726=CARTESIAN_POINT('Origin',(0.,0.,133.410000002)) ;
#11727=CARTESIAN_POINT('',(6.52951856112,-0.961970560881,132.9)) ;
#11728=CARTESIAN_POINT('Origin',(0.,0.,132.9)) ;
#11729=CARTESIAN_POINT('',(6.52951856112,-0.961970560881,132.6)) ;
#11730=CARTESIAN_POINT('Origin',(0.,0.,132.6)) ;
#11731=CARTESIAN_POINT('',(6.52951856112,-0.961970560881,133.410000002)) ;
#11732=CARTESIAN_POINT('Origin',(1.40837433338,6.75473772526,128.55)) ;
#11733=CARTESIAN_POINT('',(0.961970560881,6.52951856112,132.6)) ;
#11734=CARTESIAN_POINT('',(0.961970560881,6.52951856112,132.9)) ;
#11735=CARTESIAN_POINT('',(0.961970560881,6.52951856112,128.55)) ;
#11736=CARTESIAN_POINT('',(1.30631822227,6.26526397705,132.6)) ;
#11737=CARTESIAN_POINT('Origin',(1.40837433338,6.75473772526,132.6)) ;
#11738=CARTESIAN_POINT('',(1.30631822227,6.26526397705,124.2)) ;
#11739=CARTESIAN_POINT('',(1.30631822227,6.26526397705,128.55)) ;
#11740=CARTESIAN_POINT('',(0.908374333382,6.75473772526,124.2)) ;
#11741=CARTESIAN_POINT('Origin',(1.40837433338,6.75473772526,124.2)) ;
#11742=CARTESIAN_POINT('',(0.908374333382,6.75473772526,132.9)) ;
#11743=CARTESIAN_POINT('',(0.908374333382,6.75473772526,128.55)) ;
#11744=CARTESIAN_POINT('Origin',(1.40837433338,6.75473772526,132.9)) ;
#11745=CARTESIAN_POINT('Origin',(0.,0.,127.6)) ;
#11746=CARTESIAN_POINT('',(-1.30631822227,6.26526397705,124.2)) ;
#11747=CARTESIAN_POINT('',(-3.50650417075,5.35391711745,124.2)) ;
#11748=CARTESIAN_POINT('Origin',(0.,0.,124.2)) ;
#11749=CARTESIAN_POINT('',(-3.50650417075,5.35391711745,132.6)) ;
#11750=CARTESIAN_POINT('',(-3.50650417075,5.35391711745,128.4)) ;
#11751=CARTESIAN_POINT('',(-1.30631822227,6.26526397705,132.6)) ;
#11752=CARTESIAN_POINT('Origin',(0.,0.,132.6)) ;
#11753=CARTESIAN_POINT('',(-1.30631822227,6.26526397705,128.4)) ;
#11754=CARTESIAN_POINT('Origin',(-3.78044980909,5.77219189225,128.55)) ;
#11755=CARTESIAN_POINT('',(-3.93685094555,5.29728275935,132.6)) ;
#11756=CARTESIAN_POINT('',(-3.93685094555,5.29728275935,132.9)) ;
#11757=CARTESIAN_POINT('',(-3.93685094555,5.29728275935,128.55)) ;
#11758=CARTESIAN_POINT('Origin',(-3.78044980909,5.77219189225,132.6)) ;
#11759=CARTESIAN_POINT('',(-4.13400319968,5.41863850166,124.2)) ;
#11760=CARTESIAN_POINT('Origin',(-3.78044980909,5.77219189225,124.2)) ;
#11761=CARTESIAN_POINT('',(-4.13400319968,5.41863850166,132.9)) ;
#11762=CARTESIAN_POINT('',(-4.13400319968,5.41863850166,128.55)) ;
#11763=CARTESIAN_POINT('Origin',(-3.78044980909,5.77219189225,132.9)) ;
#11764=CARTESIAN_POINT('Origin',(0.,0.,127.6)) ;
#11765=CARTESIAN_POINT('',(-5.35391711745,3.50650417075,132.6)) ;
#11766=CARTESIAN_POINT('',(-6.26526397705,1.30631822227,132.6)) ;
#11767=CARTESIAN_POINT('Origin',(0.,0.,132.6)) ;
#11768=CARTESIAN_POINT('',(-5.35391711745,3.50650417075,124.2)) ;
#11769=CARTESIAN_POINT('',(-5.35391711745,3.50650417075,128.4)) ;
#11770=CARTESIAN_POINT('',(-6.26526397705,1.30631822227,124.2)) ;
#11771=CARTESIAN_POINT('Origin',(0.,0.,124.2)) ;
#11772=CARTESIAN_POINT('',(-6.26526397705,1.30631822227,128.4)) ;
#11773=CARTESIAN_POINT('Origin',(-6.75473772526,1.40837433338,128.55)) ;
#11774=CARTESIAN_POINT('',(-6.52951856112,0.961970560881,132.6)) ;
#11775=CARTESIAN_POINT('',(-6.52951856112,0.961970560881,132.9)) ;
#11776=CARTESIAN_POINT('',(-6.52951856112,0.961970560881,128.55)) ;
#11777=CARTESIAN_POINT('Origin',(-6.75473772526,1.40837433338,132.6)) ;
#11778=CARTESIAN_POINT('',(-6.75473772526,0.908374333382,124.2)) ;
#11779=CARTESIAN_POINT('Origin',(-6.75473772526,1.40837433338,124.2)) ;
#11780=CARTESIAN_POINT('',(-6.75473772526,0.908374333382,132.9)) ;
#11781=CARTESIAN_POINT('',(-6.75473772526,0.908374333382,128.55)) ;
#11782=CARTESIAN_POINT('Origin',(-6.75473772526,1.40837433338,132.9)) ;
#11783=CARTESIAN_POINT('Origin',(0.,0.,127.6)) ;
#11784=CARTESIAN_POINT('',(-6.26526397705,-1.30631822227,132.6)) ;
#11785=CARTESIAN_POINT('',(-5.35391711745,-3.50650417075,132.6)) ;
#11786=CARTESIAN_POINT('Origin',(0.,0.,132.6)) ;
#11787=CARTESIAN_POINT('',(-6.26526397705,-1.30631822227,124.2)) ;
#11788=CARTESIAN_POINT('',(-6.26526397705,-1.30631822227,128.4)) ;
#11789=CARTESIAN_POINT('',(-5.35391711745,-3.50650417075,124.2)) ;
#11790=CARTESIAN_POINT('Origin',(0.,0.,124.2)) ;
#11791=CARTESIAN_POINT('',(-5.35391711745,-3.50650417075,128.4)) ;
#11792=CARTESIAN_POINT('Origin',(-5.77219189225,-3.78044980909,128.55)) ;
#11793=CARTESIAN_POINT('',(-5.29728275935,-3.93685094555,132.6)) ;
#11794=CARTESIAN_POINT('',(-5.29728275935,-3.93685094555,132.9)) ;
#11795=CARTESIAN_POINT('',(-5.29728275935,-3.93685094555,128.55)) ;
#11796=CARTESIAN_POINT('Origin',(-5.77219189225,-3.78044980909,132.6)) ;
#11797=CARTESIAN_POINT('',(-5.41863850166,-4.13400319968,124.2)) ;
#11798=CARTESIAN_POINT('Origin',(-5.77219189225,-3.78044980909,124.2)) ;
#11799=CARTESIAN_POINT('',(-5.41863850166,-4.13400319968,132.9)) ;
#11800=CARTESIAN_POINT('',(-5.41863850166,-4.13400319968,128.55)) ;
#11801=CARTESIAN_POINT('Origin',(-5.77219189225,-3.78044980909,132.9)) ;
#11802=CARTESIAN_POINT('Origin',(0.,0.,127.6)) ;
#11803=CARTESIAN_POINT('',(-3.50650417075,-5.35391711745,132.6)) ;
#11804=CARTESIAN_POINT('',(-1.30631822227,-6.26526397705,132.6)) ;
#11805=CARTESIAN_POINT('Origin',(0.,0.,132.6)) ;
#11806=CARTESIAN_POINT('',(-3.50650417075,-5.35391711745,124.2)) ;
#11807=CARTESIAN_POINT('',(-3.50650417075,-5.35391711745,128.4)) ;
#11808=CARTESIAN_POINT('',(-1.30631822227,-6.26526397705,124.2)) ;
#11809=CARTESIAN_POINT('Origin',(0.,0.,124.2)) ;
#11810=CARTESIAN_POINT('',(-1.30631822227,-6.26526397705,128.4)) ;
#11811=CARTESIAN_POINT('Origin',(-1.40837433338,-6.75473772526,128.55)) ;
#11812=CARTESIAN_POINT('',(-0.961970560881,-6.52951856112,132.6)) ;
#11813=CARTESIAN_POINT('',(-0.961970560881,-6.52951856112,132.9)) ;
#11814=CARTESIAN_POINT('',(-0.961970560881,-6.52951856112,128.55)) ;
#11815=CARTESIAN_POINT('Origin',(-1.40837433338,-6.75473772526,132.6)) ;
#11816=CARTESIAN_POINT('',(-0.908374333382,-6.75473772526,124.2)) ;
#11817=CARTESIAN_POINT('Origin',(-1.40837433338,-6.75473772526,124.2)) ;
#11818=CARTESIAN_POINT('',(-0.908374333382,-6.75473772526,132.9)) ;
#11819=CARTESIAN_POINT('',(-0.908374333382,-6.75473772526,128.55)) ;
#11820=CARTESIAN_POINT('Origin',(-1.40837433338,-6.75473772526,132.9)) ;
#11821=CARTESIAN_POINT('Origin',(0.,0.,127.6)) ;
#11822=CARTESIAN_POINT('',(1.30631822227,-6.26526397705,124.2)) ;
#11823=CARTESIAN_POINT('',(3.50650417075,-5.35391711745,124.2)) ;
#11824=CARTESIAN_POINT('Origin',(0.,0.,124.2)) ;
#11825=CARTESIAN_POINT('',(3.50650417075,-5.35391711745,132.6)) ;
#11826=CARTESIAN_POINT('',(3.50650417075,-5.35391711745,128.4)) ;
#11827=CARTESIAN_POINT('',(1.30631822227,-6.26526397705,132.6)) ;
#11828=CARTESIAN_POINT('Origin',(0.,0.,132.6)) ;
#11829=CARTESIAN_POINT('',(1.30631822227,-6.26526397705,128.4)) ;
#11830=CARTESIAN_POINT('Origin',(3.78044980909,-5.77219189225,128.55)) ;
#11831=CARTESIAN_POINT('',(3.93685094555,-5.29728275935,132.6)) ;
#11832=CARTESIAN_POINT('',(3.93685094555,-5.29728275935,132.9)) ;
#11833=CARTESIAN_POINT('',(3.93685094555,-5.29728275935,128.55)) ;
#11834=CARTESIAN_POINT('Origin',(3.78044980909,-5.77219189225,132.6)) ;
#11835=CARTESIAN_POINT('',(4.13400319968,-5.41863850166,124.2)) ;
#11836=CARTESIAN_POINT('Origin',(3.78044980909,-5.77219189225,124.2)) ;
#11837=CARTESIAN_POINT('',(4.13400319968,-5.41863850166,132.9)) ;
#11838=CARTESIAN_POINT('',(4.13400319968,-5.41863850166,128.55)) ;
#11839=CARTESIAN_POINT('Origin',(3.78044980909,-5.77219189225,132.9)) ;
#11840=CARTESIAN_POINT('Origin',(0.,0.,127.6)) ;
#11841=CARTESIAN_POINT('',(5.35391711745,-3.50650417075,132.6)) ;
#11842=CARTESIAN_POINT('',(6.26526397705,-1.30631822227,132.6)) ;
#11843=CARTESIAN_POINT('Origin',(0.,0.,132.6)) ;
#11844=CARTESIAN_POINT('',(5.35391711745,-3.50650417075,124.2)) ;
#11845=CARTESIAN_POINT('',(5.35391711745,-3.50650417075,128.4)) ;
#11846=CARTESIAN_POINT('',(6.26526397705,-1.30631822227,124.2)) ;
#11847=CARTESIAN_POINT('Origin',(0.,0.,124.2)) ;
#11848=CARTESIAN_POINT('',(6.26526397705,-1.30631822227,128.4)) ;
#11849=CARTESIAN_POINT('Origin',(0.,0.,133.410000002)) ;
#11850=CARTESIAN_POINT('',(-6.52951856112,-0.961970560881,132.9)) ;
#11851=CARTESIAN_POINT('Origin',(0.,0.,132.9)) ;
#11852=CARTESIAN_POINT('',(-6.52951856112,-0.961970560881,132.6)) ;
#11853=CARTESIAN_POINT('',(-6.52951856112,-0.961970560881,133.410000002)) ;
#11854=CARTESIAN_POINT('Origin',(0.,0.,132.6)) ;
#11855=CARTESIAN_POINT('Origin',(0.,0.,133.410000002)) ;
#11856=CARTESIAN_POINT('',(5.29728275935,-3.93685094555,132.9)) ;
#11857=CARTESIAN_POINT('Origin',(0.,0.,132.9)) ;
#11858=CARTESIAN_POINT('',(5.29728275935,-3.93685094555,132.6)) ;
#11859=CARTESIAN_POINT('',(5.29728275935,-3.93685094555,133.410000002)) ;
#11860=CARTESIAN_POINT('Origin',(0.,0.,132.6)) ;
#11861=CARTESIAN_POINT('Origin',(0.,0.,133.410000002)) ;
#11862=CARTESIAN_POINT('',(0.961970560881,-6.52951856112,132.9)) ;
#11863=CARTESIAN_POINT('Origin',(0.,0.,132.9)) ;
#11864=CARTESIAN_POINT('',(0.961970560881,-6.52951856112,132.6)) ;
#11865=CARTESIAN_POINT('',(0.961970560881,-6.52951856112,133.410000002)) ;
#11866=CARTESIAN_POINT('Origin',(0.,0.,132.6)) ;
#11867=CARTESIAN_POINT('Origin',(0.,0.,133.410000002)) ;
#11868=CARTESIAN_POINT('',(-3.93685094555,-5.29728275935,132.9)) ;
#11869=CARTESIAN_POINT('Origin',(0.,0.,132.9)) ;
#11870=CARTESIAN_POINT('',(-3.93685094555,-5.29728275935,132.6)) ;
#11871=CARTESIAN_POINT('',(-3.93685094555,-5.29728275935,133.410000002)) ;
#11872=CARTESIAN_POINT('Origin',(0.,0.,132.6)) ;
#11873=CARTESIAN_POINT('Origin',(0.,0.,133.410000002)) ;
#11874=CARTESIAN_POINT('',(-5.29728275935,3.93685094555,132.9)) ;
#11875=CARTESIAN_POINT('Origin',(0.,0.,132.9)) ;
#11876=CARTESIAN_POINT('',(-5.29728275935,3.93685094555,132.6)) ;
#11877=CARTESIAN_POINT('',(-5.29728275935,3.93685094555,133.410000002)) ;
#11878=CARTESIAN_POINT('Origin',(0.,0.,132.6)) ;
#11879=CARTESIAN_POINT('Origin',(0.,0.,133.410000002)) ;
#11880=CARTESIAN_POINT('',(-0.961970560881,6.52951856112,132.9)) ;
#11881=CARTESIAN_POINT('Origin',(0.,0.,132.9)) ;
#11882=CARTESIAN_POINT('',(-0.961970560881,6.52951856112,132.6)) ;
#11883=CARTESIAN_POINT('',(-0.961970560881,6.52951856112,133.410000002)) ;
#11884=CARTESIAN_POINT('Origin',(0.,0.,132.6)) ;
#11885=CARTESIAN_POINT('Origin',(0.,0.,127.6)) ;
#11886=CARTESIAN_POINT('',(3.50650417075,5.35391711745,132.6)) ;
#11887=CARTESIAN_POINT('Origin',(0.,0.,132.6)) ;
#11888=CARTESIAN_POINT('',(3.50650417075,5.35391711745,124.2)) ;
#11889=CARTESIAN_POINT('',(3.50650417075,5.35391711745,128.4)) ;
#11890=CARTESIAN_POINT('Origin',(0.,0.,124.2)) ;
#11891=CARTESIAN_POINT('Origin',(6.75473772526,-1.40837433338,128.55)) ;
#11892=CARTESIAN_POINT('Origin',(6.75473772526,-1.40837433338,132.6)) ;
#11893=CARTESIAN_POINT('',(6.75473772526,-0.908374333382,124.2)) ;
#11894=CARTESIAN_POINT('Origin',(6.75473772526,-1.40837433338,124.2)) ;
#11895=CARTESIAN_POINT('',(6.75473772526,-0.908374333382,132.9)) ;
#11896=CARTESIAN_POINT('',(6.75473772526,-0.908374333382,128.55)) ;
#11897=CARTESIAN_POINT('Origin',(6.75473772526,-1.40837433338,132.9)) ;
#11898=CARTESIAN_POINT('Origin',(-5.77219189225,3.78044980909,128.55)) ;
#11899=CARTESIAN_POINT('Origin',(-5.77219189225,3.78044980909,132.6)) ;
#11900=CARTESIAN_POINT('Origin',(-5.77219189225,3.78044980909,132.9)) ;
#11901=CARTESIAN_POINT('Origin',(-5.77219189225,3.78044980909,124.2)) ;
#11902=CARTESIAN_POINT('Origin',(-6.75473772526,-1.40837433338,128.55)) ;
#11903=CARTESIAN_POINT('Origin',(-6.75473772526,-1.40837433338,132.6)) ;
#11904=CARTESIAN_POINT('Origin',(-6.75473772526,-1.40837433338,132.9)) ;
#11905=CARTESIAN_POINT('Origin',(-6.75473772526,-1.40837433338,124.2)) ;
#11906=CARTESIAN_POINT('Origin',(-3.78044980909,-5.77219189225,128.55)) ;
#11907=CARTESIAN_POINT('Origin',(-3.78044980909,-5.77219189225,132.6)) ;
#11908=CARTESIAN_POINT('Origin',(-3.78044980909,-5.77219189225,132.9)) ;
#11909=CARTESIAN_POINT('Origin',(-3.78044980909,-5.77219189225,124.2)) ;
#11910=CARTESIAN_POINT('Origin',(1.40837433338,-6.75473772526,128.55)) ;
#11911=CARTESIAN_POINT('Origin',(1.40837433338,-6.75473772526,132.6)) ;
#11912=CARTESIAN_POINT('Origin',(1.40837433338,-6.75473772526,132.9)) ;
#11913=CARTESIAN_POINT('Origin',(1.40837433338,-6.75473772526,124.2)) ;
#11914=CARTESIAN_POINT('Origin',(-1.40837433338,6.75473772526,128.55)) ;
#11915=CARTESIAN_POINT('Origin',(-1.40837433338,6.75473772526,132.6)) ;
#11916=CARTESIAN_POINT('Origin',(-1.40837433338,6.75473772526,132.9)) ;
#11917=CARTESIAN_POINT('Origin',(-1.40837433338,6.75473772526,124.2)) ;
#11918=CARTESIAN_POINT('Origin',(-15.2192295004,16.5038648024,124.2)) ;
#11919=CARTESIAN_POINT('',(-9.67661635003,10.961251652,124.2)) ;
#11920=CARTESIAN_POINT('',(-9.67661635003,10.961251652,132.9)) ;
#11921=CARTESIAN_POINT('Origin',(0.,0.,132.9)) ;
#11922=CARTESIAN_POINT('Origin',(0.,-22.45,124.2)) ;
#11923=CARTESIAN_POINT('',(-14.5931764135,0.908374333382,124.2)) ;
#11924=CARTESIAN_POINT('Origin',(-22.4316151017,0.908374333382,124.2)) ;
#11925=CARTESIAN_POINT('',(-14.5931764135,0.908374333382,132.9)) ;
#11926=CARTESIAN_POINT('Origin',(0.,0.,132.9)) ;
#11927=CARTESIAN_POINT('Origin',(0.,-22.45,124.2)) ;
#11928=CARTESIAN_POINT('',(-10.961251652,-9.67661635003,124.2)) ;
#11929=CARTESIAN_POINT('Origin',(-16.5038648024,-15.2192295004,124.2)) ;
#11930=CARTESIAN_POINT('',(-10.961251652,-9.67661635003,132.9)) ;
#11931=CARTESIAN_POINT('Origin',(0.,0.,132.9)) ;
#11932=CARTESIAN_POINT('Origin',(0.,-22.45,124.2)) ;
#11933=CARTESIAN_POINT('',(-0.908374333382,-14.5931764135,124.2)) ;
#11934=CARTESIAN_POINT('Origin',(-0.908374333382,-22.4316151017,124.2)) ;
#11935=CARTESIAN_POINT('',(-0.908374333382,-14.5931764135,132.9)) ;
#11936=CARTESIAN_POINT('Origin',(0.,0.,132.9)) ;
#11937=CARTESIAN_POINT('Origin',(5.77219189225,-3.78044980909,128.55)) ;
#11938=CARTESIAN_POINT('Origin',(5.77219189225,-3.78044980909,132.6)) ;
#11939=CARTESIAN_POINT('Origin',(5.77219189225,-3.78044980909,132.9)) ;
#11940=CARTESIAN_POINT('Origin',(5.77219189225,-3.78044980909,124.2)) ;
#11941=CARTESIAN_POINT('Origin',(0.,0.,127.6)) ;
#11942=CARTESIAN_POINT('',(5.35391711745,3.50650417075,132.6)) ;
#11943=CARTESIAN_POINT('Origin',(0.,0.,132.6)) ;
#11944=CARTESIAN_POINT('',(5.35391711745,3.50650417075,128.4)) ;
#11945=CARTESIAN_POINT('Origin',(0.,0.,132.9)) ;
#11946=CARTESIAN_POINT('',(0.908374333382,14.5931764135,132.9)) ;
#11947=CARTESIAN_POINT('Origin',(0.,-22.45,124.2)) ;
#11948=CARTESIAN_POINT('Origin',(0.,-22.45,124.2)) ;
#11949=CARTESIAN_POINT('',(9.67661635003,-10.961251652,124.2)) ;
#11950=CARTESIAN_POINT('Origin',(15.2192295004,-16.5038648024,124.2)) ;
#11951=CARTESIAN_POINT('',(9.67661635003,-10.961251652,132.9)) ;
#11952=CARTESIAN_POINT('Origin',(0.,0.,132.9)) ;
#11953=CARTESIAN_POINT('Origin',(0.,-22.45,124.2)) ;
#11954=CARTESIAN_POINT('',(14.5931764135,-0.908374333382,124.2)) ;
#11955=CARTESIAN_POINT('Origin',(22.4316151017,-0.908374333382,124.2)) ;
#11956=CARTESIAN_POINT('',(14.5931764135,-0.908374333382,132.9)) ;
#11957=CARTESIAN_POINT('Origin',(0.,0.,132.9)) ;
#11958=CARTESIAN_POINT('Origin',(0.,-22.45,124.2)) ;
#11959=CARTESIAN_POINT('Origin',(3.78044980909,5.77219189225,124.2)) ;
#11960=CARTESIAN_POINT('',(0.908374333382,14.5931764135,124.2)) ;
#11961=CARTESIAN_POINT('Origin',(0.908374333382,22.4316151017,124.2)) ;
#11962=CARTESIAN_POINT('Origin',(5.77219189225,3.78044980909,128.55)) ;
#11963=CARTESIAN_POINT('Origin',(5.77219189225,3.78044980909,132.6)) ;
#11964=CARTESIAN_POINT('Origin',(3.78044980909,5.77219189225,128.55)) ;
#11965=CARTESIAN_POINT('Origin',(3.78044980909,5.77219189225,132.6)) ;
#11966=CARTESIAN_POINT('Origin',(0.,-6.4,132.6)) ;
#13479=UNCERTAINTY_MEASURE_WITH_UNIT(LENGTH_MEASURE(0.01),#13511,
'DISTANCE_ACCURACY_VALUE',
'Maximum model space distance between geometric entities at asserted c
onnectivities') ;
#13493=UNCERTAINTY_MEASURE_WITH_UNIT(LENGTH_MEASURE(0.01),#13511,
'DISTANCE_ACCURACY_VALUE',
'Maximum model space distance between geometric entities at asserted c
onnectivities') ;
#13496=(
GEOMETRIC_REPRESENTATION_CONTEXT(3)
GLOBAL_UNCERTAINTY_ASSIGNED_CONTEXT((#13479))
GLOBAL_UNIT_ASSIGNED_CONTEXT((#13511,#13513,#13514))
REPRESENTATION_CONTEXT('','3D')
) ;
#13510=(
GEOMETRIC_REPRESENTATION_CONTEXT(3)
GLOBAL_UNCERTAINTY_ASSIGNED_CONTEXT((#13493))
GLOBAL_UNIT_ASSIGNED_CONTEXT((#13511,#13513,#13514))
REPRESENTATION_CONTEXT('','3D')
) ;
#13511=(
LENGTH_UNIT()
NAMED_UNIT(*)
SI_UNIT(.MILLI.,.METRE.)
) ;
#13513=(
NAMED_UNIT(*)
PLANE_ANGLE_UNIT()
SI_UNIT($,.RADIAN.)
) ;
#13514=(
NAMED_UNIT(*)
SI_UNIT($,.STERADIAN.)
SOLID_ANGLE_UNIT()
) ;
#13517=SHAPE_DEFINITION_REPRESENTATION(#13533,#13564) ;
#13533=PRODUCT_DEFINITION_SHAPE('',$,#13581) ;
#13564=SHAPE_REPRESENTATION('',(#7719),#13496) ;
#13578=PRODUCT_DEFINITION_CONTEXT('part definition',#13628,'design') ;
#13581=PRODUCT_DEFINITION('Rear_End_Cap','Rear_End_Cap',#13597,#13578) ;
#13597=PRODUCT_DEFINITION_FORMATION('',$,#13632) ;
#13628=APPLICATION_CONTEXT(
'Core Data for Automotive Mechanical Design Process') ;
#13629=PRODUCT_CONTEXT('part definition',#13628,'mechanical') ;
#13632=PRODUCT('Rear_End_Cap','Rear_End_Cap',$,(#13629)) ;
#13648=PRESENTATION_STYLE_ASSIGNMENT((#13653)) ;
#13653=SURFACE_STYLE_USAGE(.BOTH.,#13658) ;
#13658=SURFACE_SIDE_STYLE('',(#13663)) ;
#13663=SURFACE_STYLE_FILL_AREA(#13668) ;
#13668=FILL_AREA_STYLE('Opaque(255,255,255)',(#13673)) ;
#13673=FILL_AREA_STYLE_COLOUR('Opaque(255,255,255)',#13678) ;
#13678=COLOUR_RGB('Opaque(255,255,255)', 0.66274510, 0.83137255, 0.94901961) ;
ENDSEC;
END-ISO-10303-21;
